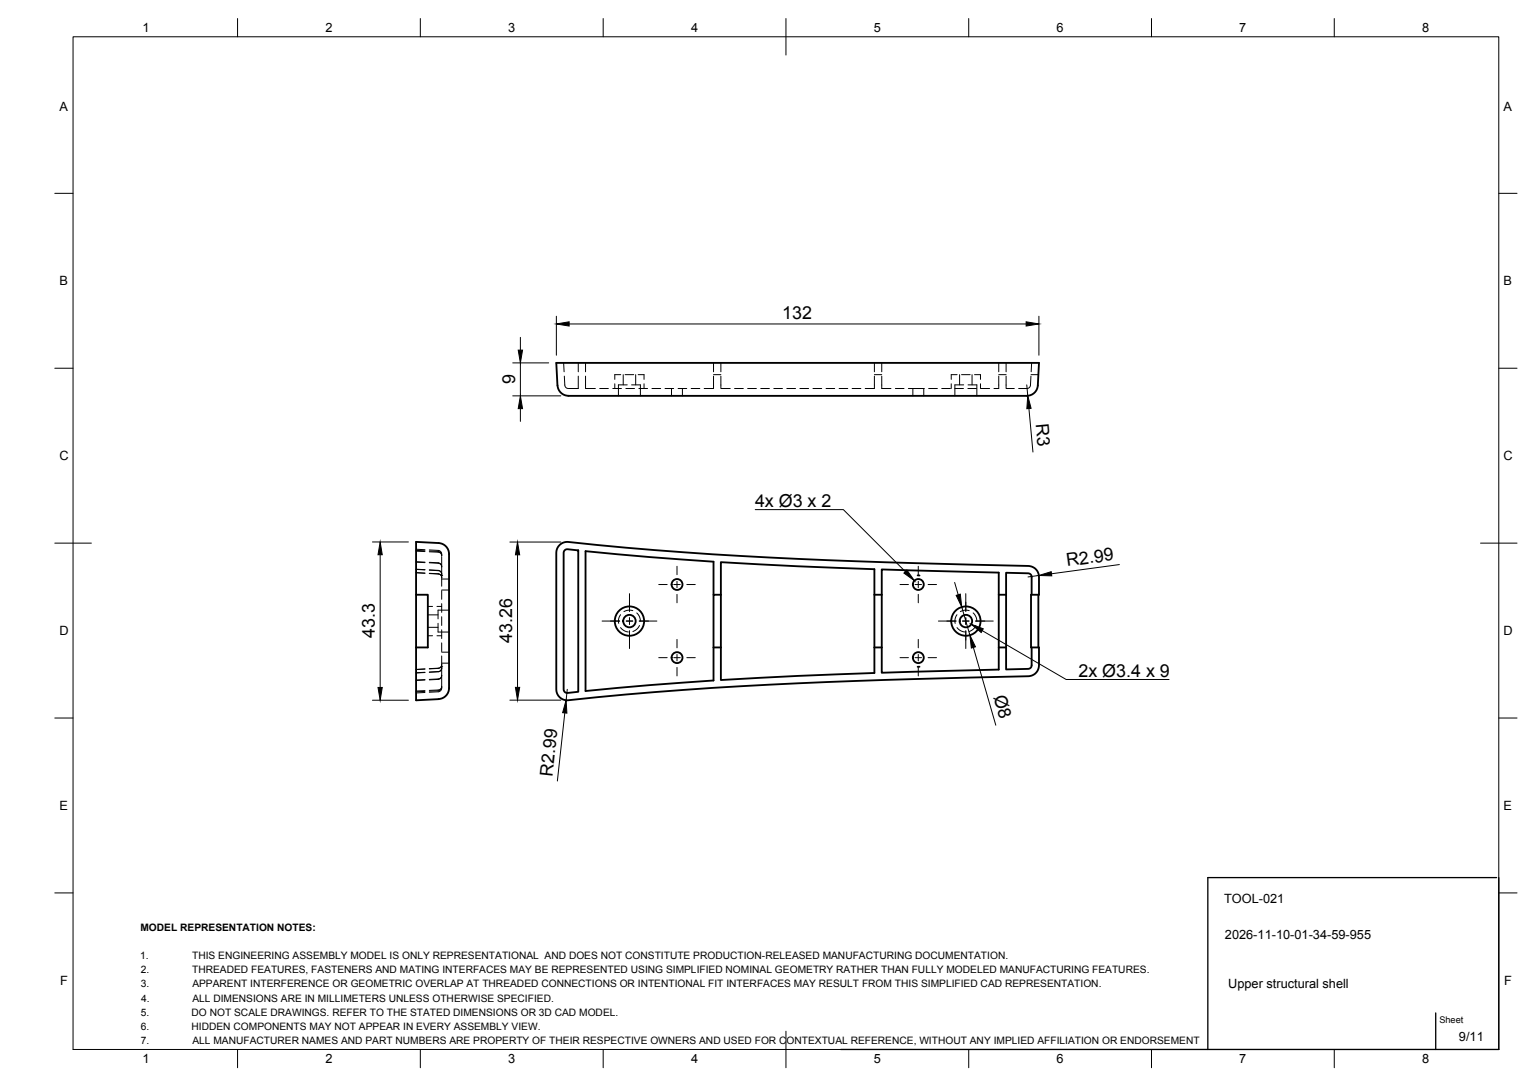
ISO-10303-21;
HEADER;
/* Generated by software containing ST-Developer
 * from STEP Tools, Inc. (www.steptools.com) 
 */

FILE_DESCRIPTION(
/* description */ (''),
/* implementation_level */ '2;1');

FILE_NAME(
/* name */ 'Upper structural shell.step',
/* time_stamp */ '2026-11-10T09:05:57-08:00',
/* author */ (''),
/* organization */ (''),
/* preprocessor_version */ 'ST-DEVELOPER v20.2',
/* originating_system */ 'Autodesk Translation Framework v15.17.0.0',
/* authorisation */ '');

FILE_SCHEMA (('AUTOMOTIVE_DESIGN { 1 0 10303 214 3 1 1 }'));
ENDSEC;

DATA;
#10=MECHANICAL_DESIGN_GEOMETRIC_PRESENTATION_REPRESENTATION('',(#569),#19618);
#75=SPHERICAL_SURFACE('',#7438,0.0999999999999999);
#76=SPHERICAL_SURFACE('',#7441,0.0999999999999997);
#77=SPHERICAL_SURFACE('',#7445,0.0999999999999998);
#78=SPHERICAL_SURFACE('',#7449,0.1);
#79=SPHERICAL_SURFACE('',#7454,0.3);
#80=SPHERICAL_SURFACE('',#7458,0.3);
#81=SPHERICAL_SURFACE('',#7462,0.3);
#82=SPHERICAL_SURFACE('',#7467,0.3);
#91=B_SPLINE_SURFACE_WITH_KNOTS('',3,3,((#10711,#10712,#10713,#10714),(#10715,
#10716,#10717,#10718),(#10719,#10720,#10721,#10722),(#10723,#10724,#10725,
#10726)),.UNSPECIFIED.,.F.,.F.,.F.,(4,4),(4,4),(0.0600191787356395,0.326709122771036),
(0.0105314009467253,0.683686938235975),.UNSPECIFIED.);
#92=B_SPLINE_SURFACE_WITH_KNOTS('',3,3,((#10731,#10732,#10733,#10734),(#10735,
#10736,#10737,#10738),(#10739,#10740,#10741,#10742),(#10743,#10744,#10745,
#10746)),.UNSPECIFIED.,.F.,.F.,.F.,(4,4),(4,4),(0.0251675824878611,0.0470055662028096),
(0.0103663370325175,0.682341693918943),.UNSPECIFIED.);
#93=B_SPLINE_SURFACE_WITH_KNOTS('',3,3,((#10756,#10757,#10758,#10759),(#10760,
#10761,#10762,#10763),(#10764,#10765,#10766,#10767),(#10768,#10769,#10770,
#10771),(#10772,#10773,#10774,#10775)),.UNSPECIFIED.,.F.,.F.,.F.,(4,1,4),
(4,4),(0.,0.571428571428571,1.),(0.796205213256333,4.31873271634551),
 .UNSPECIFIED.);
#94=B_SPLINE_SURFACE_WITH_KNOTS('',3,3,((#10780,#10781,#10782,#10783),(#10784,
#10785,#10786,#10787),(#10788,#10789,#10790,#10791),(#10792,#10793,#10794,
#10795),(#10796,#10797,#10798,#10799)),.UNSPECIFIED.,.F.,.F.,.F.,(4,1,4),
(4,4),(0.,0.571428571428571,1.),(0.335767855111383,0.605460332260614),
 .UNSPECIFIED.);
#95=B_SPLINE_SURFACE_WITH_KNOTS('',3,3,((#10818,#10819,#10820,#10821),(#10822,
#10823,#10824,#10825),(#10826,#10827,#10828,#10829),(#10830,#10831,#10832,
#10833),(#10834,#10835,#10836,#10837)),.UNSPECIFIED.,.F.,.F.,.F.,(4,1,4),
(4,4),(0.,0.571428571428571,1.),(8.8675541747208,12.3900816778099),
 .UNSPECIFIED.);
#96=B_SPLINE_SURFACE_WITH_KNOTS('',3,3,((#10842,#10843,#10844,#10845),(#10846,
#10847,#10848,#10849),(#10850,#10851,#10852,#10853),(#10854,#10855,#10856,
#10857)),.UNSPECIFIED.,.F.,.F.,.F.,(4,4),(4,4),(0.673290877228964,0.939980821264432),
(0.010531400969624,0.683686938235975),.UNSPECIFIED.);
#97=B_SPLINE_SURFACE_WITH_KNOTS('',3,3,((#10858,#10859,#10860,#10861),(#10862,
#10863,#10864,#10865),(#10866,#10867,#10868,#10869),(#10870,#10871,#10872,
#10873)),.UNSPECIFIED.,.F.,.F.,.F.,(4,4),(4,4),(0.952994433797115,0.974832417512139),
(0.0103663370325174,0.682341693895801),.UNSPECIFIED.);
#98=B_SPLINE_SURFACE_WITH_KNOTS('',3,3,((#10957,#10958,#10959,#10960),(#10961,
#10962,#10963,#10964),(#10965,#10966,#10967,#10968),(#10969,#10970,#10971,
#10972)),.UNSPECIFIED.,.F.,.F.,.F.,(4,4),(4,4),(0.341076481775573,0.660379921919131),
(0.0113804342297301,0.684288445414502),.UNSPECIFIED.);
#99=B_SPLINE_SURFACE_WITH_KNOTS('',3,3,((#10977,#10978,#10979,#10980),(#10981,
#10982,#10983,#10984),(#10985,#10986,#10987,#10988),(#10989,#10990,#10991,
#10992),(#10993,#10994,#10995,#10996)),.UNSPECIFIED.,.F.,.F.,.F.,(4,1,4),
(4,4),(0.,0.571428571428571,1.),(4.5128966022766,8.72381854299666),
 .UNSPECIFIED.);
#100=B_SPLINE_SURFACE_WITH_KNOTS('',3,3,((#11006,#11007,#11008,#11009),
(#11010,#11011,#11012,#11013),(#11014,#11015,#11016,#11017),(#11018,#11019,
#11020,#11021),(#11022,#11023,#11024,#11025)),.UNSPECIFIED.,.F.,.F.,.F.,
(4,1,4),(4,4),(0.,0.571428571428571,1.),(4.46246834806959,8.67339028878965),
 .UNSPECIFIED.);
#101=B_SPLINE_SURFACE_WITH_KNOTS('',3,3,((#11030,#11031,#11032,#11033),
(#11034,#11035,#11036,#11037),(#11038,#11039,#11040,#11041),(#11042,#11043,
#11044,#11045)),.UNSPECIFIED.,.F.,.F.,.F.,(4,4),(4,4),(0.33962007808087,
0.658923518224427),(0.0113804342297301,0.68428844541339),.UNSPECIFIED.);
#102=B_SPLINE_SURFACE_WITH_KNOTS('',3,3,((#11117,#11118,#11119,#11120),
(#11121,#11122,#11123,#11124),(#11125,#11126,#11127,#11128),(#11129,#11130,
#11131,#11132)),.UNSPECIFIED.,.F.,.F.,.F.,(4,4),(4,4),(0.67474627241906,
0.91907102854965),(0.0117551961069005,0.684448842095107),.UNSPECIFIED.);
#103=B_SPLINE_SURFACE_WITH_KNOTS('',3,3,((#11137,#11138,#11139,#11140),
(#11141,#11142,#11143,#11144),(#11145,#11146,#11147,#11148),(#11149,#11150,
#11151,#11152),(#11153,#11154,#11155,#11156)),.UNSPECIFIED.,.F.,.F.,.F.,
(4,1,4),(4,4),(0.,0.571428571428571,1.),(8.92068531110742,12.1251256661408),
 .UNSPECIFIED.);
#104=B_SPLINE_SURFACE_WITH_KNOTS('',3,3,((#11157,#11158,#11159,#11160),
(#11161,#11162,#11163,#11164),(#11165,#11166,#11167,#11168),(#11169,#11170,
#11171,#11172),(#11173,#11174,#11175,#11176)),.UNSPECIFIED.,.F.,.F.,.F.,
(4,1,4),(4,4),(0.,0.571428571428571,1.),(1.06116122492545,4.26560157995882),
 .UNSPECIFIED.);
#105=B_SPLINE_SURFACE_WITH_KNOTS('',3,3,((#11181,#11182,#11183,#11184),
(#11185,#11186,#11187,#11188),(#11189,#11190,#11191,#11192),(#11193,#11194,
#11195,#11196)),.UNSPECIFIED.,.F.,.F.,.F.,(4,4),(4,4),(0.0809289714503497,
0.325253727580939),(0.011755196108102,0.684448842095106),.UNSPECIFIED.);
#106=B_SPLINE_SURFACE_WITH_KNOTS('',3,3,((#11271,#11272,#11273,#11274),
(#11275,#11276,#11277,#11278),(#11279,#11280,#11281,#11282),(#11283,#11284,
#11285,#11286)),.UNSPECIFIED.,.F.,.F.,.F.,(4,4),(4,4),(0.932204931312898,
0.977820042778932),(0.0118590921259657,0.68448768567755),.UNSPECIFIED.);
#107=B_SPLINE_SURFACE_WITH_KNOTS('',3,3,((#11296,#11297,#11298,#11299),
(#11300,#11301,#11302,#11303),(#11304,#11305,#11306,#11307),(#11308,#11309,
#11310,#11311),(#11312,#11313,#11314,#11315)),.UNSPECIFIED.,.F.,.F.,.F.,
(4,1,4),(4,4),(0.,0.571428571428571,1.),(12.3228618033436,12.893479658151),
 .UNSPECIFIED.);
#108=B_SPLINE_SURFACE_WITH_KNOTS('',3,3,((#11329,#11330,#11331,#11332),
(#11333,#11334,#11335,#11336),(#11337,#11338,#11339,#11340),(#11341,#11342,
#11343,#11344)),.UNSPECIFIED.,.F.,.F.,.F.,(4,4),(4,4),(0.0221799572210682,
0.0677950686870383),(0.0118590921467069,0.68448768567755),.UNSPECIFIED.);
#109=B_SPLINE_SURFACE_WITH_KNOTS('',3,3,((#11354,#11355,#11356,#11357),
(#11358,#11359,#11360,#11361),(#11362,#11363,#11364,#11365),(#11366,#11367,
#11368,#11369),(#11370,#11371,#11372,#11373)),.UNSPECIFIED.,.F.,.F.,.F.,
(4,1,4),(4,4),(0.,0.571428571428571,1.),(0.29280723291527,0.863425087722636),
 .UNSPECIFIED.);
#110=B_SPLINE_SURFACE_WITH_KNOTS('',3,3,((#11387,#11388,#11389,#11390),
(#11391,#11392,#11393,#11394),(#11395,#11396,#11397,#11398),(#11399,#11400,
#11401,#11402),(#11403,#11404,#11405,#11406)),.UNSPECIFIED.,.F.,.F.,.F.,
(4,1,4),(4,4),(0.,0.571428571428571,1.),(0.00866835330220971,0.617725317592517),
 .UNSPECIFIED.);
#111=B_SPLINE_SURFACE_WITH_KNOTS('',3,3,((#11413,#11414,#11415,#11416),
(#11417,#11418,#11419,#11420),(#11421,#11422,#11423,#11424),(#11425,#11426,
#11427,#11428),(#11429,#11430,#11431,#11432),(#11433,#11434,#11435,#11436)),
 .UNSPECIFIED.,.F.,.F.,.F.,(4,1,1,4),(4,4),(0.,0.285714285714286,0.571428571428571,
1.),(0.00654045782928703,0.615688454110788),.UNSPECIFIED.);
#112=B_SPLINE_SURFACE_WITH_KNOTS('',3,3,((#11441,#11442,#11443,#11444),
(#11445,#11446,#11447,#11448),(#11449,#11450,#11451,#11452),(#11453,#11454,
#11455,#11456),(#11457,#11458,#11459,#11460),(#11461,#11462,#11463,#11464)),
 .UNSPECIFIED.,.F.,.F.,.F.,(4,1,1,4),(4,4),(0.,0.285714285714286,0.571428571428571,
1.),(0.00659363931523289,0.615688454110787),.UNSPECIFIED.);
#113=B_SPLINE_SURFACE_WITH_KNOTS('',3,3,((#11469,#11470,#11471,#11472),
(#11473,#11474,#11475,#11476),(#11477,#11478,#11479,#11480),(#11481,#11482,
#11483,#11484),(#11485,#11486,#11487,#11488)),.UNSPECIFIED.,.F.,.F.,.F.,
(4,1,4),(4,4),(0.,0.571428571428571,1.),(12.5808265588057,12.8505190359549),
 .UNSPECIFIED.);
#114=B_SPLINE_SURFACE_WITH_KNOTS('',3,3,((#11489,#11490,#11491,#11492),
(#11493,#11494,#11495,#11496),(#11497,#11498,#11499,#11500),(#11501,#11502,
#11503,#11504),(#11505,#11506,#11507,#11508)),.UNSPECIFIED.,.F.,.F.,.F.,
(4,1,4),(4,4),(0.,0.571428571428571,1.),(0.00865878607617127,0.617725317592517),
 .UNSPECIFIED.);
#115=B_SPLINE_SURFACE_WITH_KNOTS('',3,3,((#11534,#11535,#11536,#11537),
(#11538,#11539,#11540,#11541),(#11542,#11543,#11544,#11545),(#11546,#11547,
#11548,#11549),(#11550,#11551,#11552,#11553)),.UNSPECIFIED.,.F.,.F.,.F.,
(4,1,4),(4,4),(0.,0.571428571428571,1.),(-0.00615755989250974,0.617725317592517),
 .UNSPECIFIED.);
#116=B_SPLINE_SURFACE_WITH_KNOTS('',3,3,((#11572,#11573,#11574,#11575,#11576),
(#11577,#11578,#11579,#11580,#11581),(#11582,#11583,#11584,#11585,#11586),
(#11587,#11588,#11589,#11590,#11591),(#11592,#11593,#11594,#11595,#11596)),
 .UNSPECIFIED.,.F.,.F.,.F.,(4,1,4),(4,1,4),(0.,0.571428571428571,1.),(0.335767855111383,
5.71764434212835,12.893479658151),.UNSPECIFIED.);
#117=B_SPLINE_SURFACE_WITH_KNOTS('',3,3,((#11607,#11608,#11609,#11610),
(#11611,#11612,#11613,#11614),(#11615,#11616,#11617,#11618),(#11619,#11620,
#11621,#11622),(#11623,#11624,#11625,#11626),(#11627,#11628,#11629,#11630)),
 .UNSPECIFIED.,.F.,.F.,.F.,(4,1,1,4),(4,4),(0.,0.285714285714286,0.571428571428571,
1.),(-0.00844595120920508,0.615688454110788),.UNSPECIFIED.);
#118=B_SPLINE_SURFACE_WITH_KNOTS('',3,3,((#11639,#11640,#11641,#11642),
(#11643,#11644,#11645,#11646),(#11647,#11648,#11649,#11650),(#11651,#11652,
#11653,#11654),(#11655,#11656,#11657,#11658),(#11659,#11660,#11661,#11662)),
 .UNSPECIFIED.,.F.,.F.,.F.,(4,1,1,4),(4,4),(0.,0.285714285714286,0.571428571428571,
1.),(-0.00828643285111643,0.615688454110787),.UNSPECIFIED.);
#119=B_SPLINE_SURFACE_WITH_KNOTS('',3,3,((#11671,#11672,#11673,#11674,#11675),
(#11676,#11677,#11678,#11679,#11680),(#11681,#11682,#11683,#11684,#11685),
(#11686,#11687,#11688,#11689,#11690),(#11691,#11692,#11693,#11694,#11695)),
 .UNSPECIFIED.,.F.,.F.,.F.,(4,1,4),(4,1,4),(0.,0.571428571428571,1.),(0.29280723291527,
7.4686425489379,12.8505190359549),.UNSPECIFIED.);
#120=B_SPLINE_SURFACE_WITH_KNOTS('',3,3,((#11706,#11707,#11708,#11709),
(#11710,#11711,#11712,#11713),(#11714,#11715,#11716,#11717),(#11718,#11719,
#11720,#11721),(#11722,#11723,#11724,#11725)),.UNSPECIFIED.,.F.,.F.,.F.,
(4,1,4),(4,4),(0.,0.571428571428571,1.),(-0.0061862132014275,0.617725317592517),
 .UNSPECIFIED.);
#121=B_SPLINE_SURFACE_WITH_KNOTS('',3,3,((#11734,#11735,#11736,#11737),
(#11738,#11739,#11740,#11741),(#11742,#11743,#11744,#11745),(#11746,#11747,
#11748,#11749)),.UNSPECIFIED.,.F.,.F.,.F.,(4,4),(4,4),(0.025165545222094,
0.977821881680028),(0.,0.68448768567755),.UNSPECIFIED.);
#122=B_SPLINE_SURFACE_WITH_KNOTS('',3,3,((#11752,#11753,#11754,#11755),
(#11756,#11757,#11758,#11759),(#11760,#11761,#11762,#11763),(#11764,#11765,
#11766,#11767)),.UNSPECIFIED.,.F.,.F.,.F.,(4,4),(4,4),(0.0221781183199723,
0.974834454777906),(0.,0.68448768567755),.UNSPECIFIED.);
#171=B_SPLINE_CURVE_WITH_KNOTS('',3,(#9725,#9726,#9727,#9728),
 .UNSPECIFIED.,.F.,.F.,(4,4),(3.28016616408593,4.26236080300681),
 .UNSPECIFIED.);
#172=B_SPLINE_CURVE_WITH_KNOTS('',3,(#9732,#9733,#9734,#9735),
 .UNSPECIFIED.,.F.,.F.,(4,4),(8.92392608805945,9.90612072688831),
 .UNSPECIFIED.);
#173=B_SPLINE_CURVE_WITH_KNOTS('',3,(#9737,#9738,#9739,#9740,#9741,#9742,
#9743,#9744,#9745,#9746,#9747,#9748,#9749,#9750,#9751,#9752,#9753,#9754,
#9755),.UNSPECIFIED.,.F.,.F.,(4,3,3,3,3,3,4),(-0.050768112872884,-0.0388528786649772,
-0.0311058171716578,-0.0259830388669653,-0.0210744122964195,-0.0143837148934404,
0.),.UNSPECIFIED.);
#174=B_SPLINE_CURVE_WITH_KNOTS('',3,(#9757,#9758,#9759,#9760),
 .UNSPECIFIED.,.F.,.F.,(4,4),(9.9568018127159,12.1251256661408),
 .UNSPECIFIED.);
#175=B_SPLINE_CURVE_WITH_KNOTS('',3,(#9764,#9765,#9766,#9767),
 .UNSPECIFIED.,.F.,.F.,(4,4),(1.06116122492545,3.22948508825557),
 .UNSPECIFIED.);
#176=B_SPLINE_CURVE_WITH_KNOTS('',3,(#9768,#9769,#9770,#9771,#9772,#9773,
#9774,#9775,#9776,#9777,#9778,#9779,#9780,#9781,#9782,#9783,#9784,#9785,
#9786),.UNSPECIFIED.,.F.,.F.,(4,3,3,3,3,3,4),(-0.0507681129736439,-0.0388528772897764,
-0.0311058147321604,-0.0259830361493327,-0.0210744097201194,-0.0143837130754026,
-9.90506278315E-9),.UNSPECIFIED.);
#177=B_SPLINE_CURVE_WITH_KNOTS('',3,(#9934,#9935,#9936,#9937,#9938,#9939),
 .UNSPECIFIED.,.F.,.F.,(4,2,4),(-0.605566356596631,-0.303329629920269,-0.000148729590407126),
 .UNSPECIFIED.);
#178=B_SPLINE_CURVE_WITH_KNOTS('',3,(#9941,#9942,#9943,#9944,#9945,#9946,
#9947,#9948,#9949,#9950,#9951,#9952,#9953,#9954,#9955,#9956,#9957,#9958,
#9959,#9960,#9961,#9962,#9963,#9964,#9965,#9966,#9967,#9968),
 .UNSPECIFIED.,.F.,.F.,(4,3,3,3,3,3,3,3,3,4),(-0.153210533292091,-0.129383071834804,
-0.117098895005168,-0.0931297672424715,-0.0778761857300216,-0.065564095006876,
-0.0417435583396367,-0.038874550231651,-0.0150983388519663,0.),
 .UNSPECIFIED.);
#179=B_SPLINE_CURVE_WITH_KNOTS('',3,(#9972,#9973,#9974,#9975,#9976,#9977,
#9978,#9979,#9980,#9981,#9982,#9983,#9984,#9985,#9986,#9987,#9988,#9989,
#9990,#9991,#9992,#9993,#9994,#9995,#9996,#9997,#9998,#9999),
 .UNSPECIFIED.,.F.,.F.,(4,3,3,3,3,3,3,3,3,4),(-0.153244081227051,-0.129493605146206,
-0.117970006482883,-0.0941492904140308,-0.0876825809854227,-0.078828741443105,
-0.0548877675055393,-0.0394694906046094,-0.0155984926894347,0.),
 .UNSPECIFIED.);
#180=B_SPLINE_CURVE_WITH_KNOTS('',3,(#10000,#10001,#10002,#10003,#10004,
#10005),.UNSPECIFIED.,.F.,.F.,(4,2,4),(-0.606539490527658,-0.303329031627741,
-0.00112184825655631),.UNSPECIFIED.);
#181=B_SPLINE_CURVE_WITH_KNOTS('',3,(#10010,#10011,#10012,#10013,#10014,
#10015),.UNSPECIFIED.,.F.,.F.,(4,2,4),(-0.606785247764818,-0.303663188081886,
-0.00088649083675002),.UNSPECIFIED.);
#182=B_SPLINE_CURVE_WITH_KNOTS('',3,(#10017,#10018,#10019,#10020,#10021,
#10022,#10023,#10024,#10025,#10026,#10027,#10028,#10029,#10030,#10031,#10032,
#10033,#10034,#10035,#10036,#10037,#10038,#10039,#10040,#10041,#10042,#10043,
#10044),.UNSPECIFIED.,.F.,.F.,(4,3,3,3,3,3,3,3,3,4),(-0.15258577077829,
-0.128839317352572,-0.117158786685373,-0.0932148261566644,-0.0780319390000633,
-0.0653676349965338,-0.0415665498371782,-0.0389909618069961,-0.0152059030050533,
0.),.UNSPECIFIED.);
#183=B_SPLINE_CURVE_WITH_KNOTS('',3,(#10048,#10049,#10050,#10051,#10052,
#10053,#10054,#10055,#10056,#10057,#10058,#10059,#10060,#10061,#10062,#10063,
#10064,#10065,#10066,#10067,#10068,#10069,#10070,#10071,#10072,#10073,#10074,
#10075),.UNSPECIFIED.,.F.,.F.,(4,3,3,3,3,3,3,3,3,4),(-0.152596853546747,
-0.128825864440686,-0.115507515430042,-0.0917263797372463,-0.0872428123353572,
-0.0783995504057471,-0.0544835945915644,-0.0392209901554083,-0.0154275313391792,
0.),.UNSPECIFIED.);
#184=B_SPLINE_CURVE_WITH_KNOTS('',3,(#10077,#10078,#10079,#10080,#10081,
#10082),.UNSPECIFIED.,.F.,.F.,(4,2,4),(-0.606440835737524,-0.303663090452391,
-0.000542069086802599),.UNSPECIFIED.);
#185=B_SPLINE_CURVE_WITH_KNOTS('',3,(#10088,#10089,#10090,#10091,#10092,
#10093),.UNSPECIFIED.,.F.,.F.,(4,2,4),(-0.607379220946441,-0.303761646676304,
-0.00124422999587004),.UNSPECIFIED.);
#186=B_SPLINE_CURVE_WITH_KNOTS('',3,(#10095,#10096,#10097,#10098,#10099,
#10100,#10101,#10102,#10103,#10104,#10105,#10106,#10107,#10108,#10109,#10110,
#10111,#10112,#10113,#10114,#10115,#10116,#10117,#10118,#10119,#10120,#10121,
#10122),.UNSPECIFIED.,.F.,.F.,(4,3,3,3,3,3,3,3,3,4),(-0.152287640102895,
-0.128554450486317,-0.115193035178751,-0.0912770810520543,-0.0781028969167454,
-0.0652733399726575,-0.0414820896655672,-0.0390446621366508,-0.0152552334863041,
0.),.UNSPECIFIED.);
#187=B_SPLINE_CURVE_WITH_KNOTS('',3,(#10126,#10127,#10128,#10129,#10130,
#10131,#10132,#10133,#10134,#10135,#10136,#10137,#10138,#10139,#10140,#10141,
#10142,#10143,#10144,#10145,#10146,#10147,#10148,#10149,#10150,#10151,#10152,
#10153),.UNSPECIFIED.,.F.,.F.,(4,3,3,3,3,3,3,3,3,4),(-0.152291020205185,
-0.128517753946702,-0.115248901231919,-0.0914807886786037,-0.0870359119466785,
-0.0782017654295232,-0.054298407767766,-0.03910658747416,-0.0153486482327859,
0.),.UNSPECIFIED.);
#188=B_SPLINE_CURVE_WITH_KNOTS('',3,(#10155,#10156,#10157,#10158,#10159,
#10160),.UNSPECIFIED.,.F.,.F.,(4,2,4),(-0.606279550122448,-0.303761677523001,
-0.000144559171857295),.UNSPECIFIED.);
#189=B_SPLINE_CURVE_WITH_KNOTS('',3,(#10166,#10167,#10168,#10169,#10170,
#10171),.UNSPECIFIED.,.F.,.F.,(4,2,4),(-0.607536685592867,-0.303784463250135,
-0.00133982193348342),.UNSPECIFIED.);
#190=B_SPLINE_CURVE_WITH_KNOTS('',3,(#10172,#10173,#10174,#10175,#10176,
#10177,#10178,#10179,#10180,#10181,#10182,#10183,#10184,#10185,#10186,#10187,
#10188,#10189,#10190,#10191,#10192,#10193,#10194,#10195,#10196,#10197,#10198,
#10199),.UNSPECIFIED.,.F.,.F.,(4,3,3,3,3,3,3,3,3,4),(-0.152217684890348,
-0.128490376540845,-0.11516578527262,-0.091253137134092,-0.0781160865160423,
-0.0652495101170982,-0.0414606291875136,-0.0390546905501479,-0.015263466236765,
0.),.UNSPECIFIED.);
#191=B_SPLINE_CURVE_WITH_KNOTS('',3,(#10201,#10202,#10203,#10204,#10205,
#10206,#10207,#10208,#10209,#10210,#10211,#10212,#10213,#10214,#10215,#10216,
#10217,#10218,#10219,#10220,#10221,#10222,#10223,#10224,#10225,#10226,#10227,
#10228),.UNSPECIFIED.,.F.,.F.,(4,3,3,3,3,3,3,3,3,4),(-0.152219351639196,
-0.128444680332832,-0.115193337419806,-0.0914284185691762,-0.0869890032859244,
-0.0781648487722283,-0.0542647883944502,-0.0390852411900305,-0.0153331469286526,
0.),.UNSPECIFIED.);
#192=B_SPLINE_CURVE_WITH_KNOTS('',3,(#10230,#10231,#10232,#10233,#10234,
#10235),.UNSPECIFIED.,.F.,.F.,(4,2,4),(-0.606231877025315,-0.303784501204342,
-3.50089943914611E-5),.UNSPECIFIED.);
#193=B_SPLINE_CURVE_WITH_KNOTS('',3,(#10241,#10242,#10243,#10244),
 .UNSPECIFIED.,.F.,.F.,(4,4),(0.0108333608245492,0.617725317592517),
 .UNSPECIFIED.);
#194=B_SPLINE_CURVE_WITH_KNOTS('',3,(#10248,#10249,#10250,#10251),
 .UNSPECIFIED.,.F.,.F.,(4,4),(-0.617725317592517,-0.0108333608245492),
 .UNSPECIFIED.);
#195=B_SPLINE_CURVE_WITH_KNOTS('',3,(#10254,#10255,#10256,#10257),
 .UNSPECIFIED.,.F.,.F.,(4,4),(8.65483889175297,12.1899094612697),
 .UNSPECIFIED.);
#196=B_SPLINE_CURVE_WITH_KNOTS('',3,(#10258,#10259,#10260,#10261),
 .UNSPECIFIED.,.F.,.F.,(4,4),(0.491886782059505,4.00844302274363),
 .UNSPECIFIED.);
#197=B_SPLINE_CURVE_WITH_KNOTS('',3,(#10264,#10265,#10266,#10267,#10268,
#10269,#10270,#10271,#10272,#10273),.UNSPECIFIED.,.F.,.F.,(4,3,3,4),(4.20909064274042,
6.3236533433415,8.26419514194387,8.41669725637478),.UNSPECIFIED.);
#198=B_SPLINE_CURVE_WITH_KNOTS('',3,(#10276,#10277,#10278,#10279),
 .UNSPECIFIED.,.F.,.F.,(4,4),(8.61714174069208,11.8187712274298),
 .UNSPECIFIED.);
#199=B_SPLINE_CURVE_WITH_KNOTS('',3,(#10283,#10284,#10285,#10286),
 .UNSPECIFIED.,.F.,.F.,(4,4),(12.0182076143484,12.6179302061492),
 .UNSPECIFIED.);
#200=B_SPLINE_CURVE_WITH_KNOTS('',3,(#10287,#10288,#10289,#10290,#10291,
#10292,#10293,#10294,#10295,#10296,#10297,#10298,#10299,#10300,#10301,#10302,
#10303,#10304,#10305,#10306,#10307,#10308,#10309,#10310,#10311,#10312,#10313,
#10314),.UNSPECIFIED.,.F.,.F.,(4,3,3,3,3,3,3,3,3,4),(0.,0.023812730958415,
0.0390943730497349,0.0628727645281949,0.0664866407211859,0.0780895647789142,
0.102003044086093,0.117056568347941,0.14081843048439,0.155095961761698),
 .UNSPECIFIED.);
#201=B_SPLINE_CURVE_WITH_KNOTS('',3,(#10318,#10319,#10320,#10321,#10322,
#10323,#10324,#10325,#10326,#10327,#10328,#10329,#10330,#10331,#10332,#10333,
#10334,#10335,#10336,#10337,#10338,#10339,#10340,#10341,#10342,#10343,#10344,
#10345,#10346,#10347,#10348,#10349,#10350,#10351,#10352,#10353,#10354),
 .UNSPECIFIED.,.F.,.F.,(4,3,3,3,3,3,3,3,3,3,3,3,4),(0.,0.0535193130531386,
0.107740084455895,0.117281563739951,0.171478196787188,0.199460035548543,
0.234266327019636,0.287962832542679,0.34249270416273,0.351167719367162,
0.408228095477446,0.46132246935065,0.46528847158773),.UNSPECIFIED.);
#202=B_SPLINE_CURVE_WITH_KNOTS('',3,(#10356,#10357,#10358,#10359),
 .UNSPECIFIED.,.F.,.F.,(4,4),(0.0221781183199723,0.974834454777906),
 .UNSPECIFIED.);
#203=B_SPLINE_CURVE_WITH_KNOTS('',3,(#10361,#10362,#10363,#10364,#10365,
#10366,#10367,#10368,#10369,#10370,#10371,#10372,#10373,#10374,#10375,#10376,
#10377,#10378,#10379,#10380,#10381,#10382,#10383,#10384,#10385,#10386,#10387,
#10388,#10389,#10390,#10391,#10392,#10393,#10394,#10395,#10396,#10397,#10398,
#10399,#10400,#10401,#10402,#10403),.UNSPECIFIED.,.F.,.F.,(4,3,3,3,3,3,
3,3,3,3,3,3,3,3,4),(0.,0.0533317239385299,0.107762434368039,0.117305236535198,
0.171635266834242,0.216430402805854,0.234303130921432,0.288010415584935,
0.341932185058889,0.351200358601802,0.360578786332496,0.414653942238971,
0.427906071157934,0.482008506259547,0.504658879840573),.UNSPECIFIED.);
#204=B_SPLINE_CURVE_WITH_KNOTS('',3,(#10407,#10408,#10409,#10410,#10411,
#10412,#10413,#10414,#10415,#10416,#10417,#10418,#10419,#10420,#10421,#10422,
#10423,#10424,#10425,#10426,#10427,#10428,#10429,#10430,#10431,#10432,#10433,
#10434,#10435,#10436,#10437,#10438,#10439,#10440,#10441,#10442,#10443,#10444,
#10445,#10446,#10447,#10448,#10449),.UNSPECIFIED.,.F.,.F.,(4,3,3,3,3,3,
3,3,3,3,3,3,3,3,4),(0.,0.0533492049661439,0.107791770949794,0.117401360885473,
0.171729175646356,0.216477851539682,0.234467324023732,0.288191829779795,
0.342104640447882,0.351366010290958,0.360619117109406,0.414688080797906,
0.427993719046535,0.482081475021072,0.504664253934307),.UNSPECIFIED.);
#205=B_SPLINE_CURVE_WITH_KNOTS('',3,(#10451,#10452,#10453,#10454),
 .UNSPECIFIED.,.F.,.F.,(4,4),(0.0251655452220943,0.977821881680028),
 .UNSPECIFIED.);
#206=B_SPLINE_CURVE_WITH_KNOTS('',3,(#10456,#10457,#10458,#10459,#10460,
#10461,#10462,#10463,#10464,#10465,#10466,#10467,#10468,#10469,#10470,#10471,
#10472,#10473,#10474,#10475,#10476,#10477,#10478,#10479,#10480,#10481,#10482,
#10483,#10484,#10485,#10486,#10487,#10488,#10489,#10490,#10491,#10492),
 .UNSPECIFIED.,.F.,.F.,(4,3,3,3,3,3,3,3,3,3,3,3,4),(0.,0.053523079491772,
0.107745541051727,0.117301531762597,0.171497090450284,0.19946878868074,
0.234298606923062,0.287998861062908,0.34252758042597,0.351197710209308,
0.408243668718811,0.4613343165756,0.465289627228313),.UNSPECIFIED.);
#207=B_SPLINE_CURVE_WITH_KNOTS('',3,(#10495,#10496,#10497,#10498,#10499,
#10500,#10501,#10502,#10503,#10504,#10505,#10506,#10507,#10508,#10509,#10510,
#10511,#10512,#10513,#10514,#10515,#10516,#10517,#10518,#10519,#10520,#10521,
#10522),.UNSPECIFIED.,.F.,.F.,(4,3,3,3,3,3,3,3,3,4),(0.,0.0238139464176845,
0.039101051769884,0.0628789982206146,0.0664894862143964,0.0781003874493316,
0.102014483019035,0.11706667068295,0.140827139970411,0.155096347075245),
 .UNSPECIFIED.);
#208=B_SPLINE_CURVE_WITH_KNOTS('',3,(#10524,#10525,#10526,#10527),
 .UNSPECIFIED.,.F.,.F.,(4,4),(2.42791692093292E-5,0.602904494019558),
 .UNSPECIFIED.);
#209=B_SPLINE_CURVE_WITH_KNOTS('',3,(#10530,#10531,#10532,#10533),
 .UNSPECIFIED.,.F.,.F.,(4,4),(0.8033909285608,4.02187648095927),
 .UNSPECIFIED.);
#210=B_SPLINE_CURVE_WITH_KNOTS('',3,(#10536,#10537,#10538,#10539,#10540,
#10541,#10542,#10543,#10544,#10545),.UNSPECIFIED.,.F.,.F.,(4,3,3,4),(4.22337623295021,
6.17414866693447,6.32726315261627,8.45313487255185),.UNSPECIFIED.);
#211=B_SPLINE_CURVE_WITH_KNOTS('',3,(#10549,#10550,#10551,#10552),
 .UNSPECIFIED.,.F.,.F.,(4,4),(12.3921295467468,12.6843586902602),
 .UNSPECIFIED.);
#212=B_SPLINE_CURVE_WITH_KNOTS('',3,(#10554,#10555,#10556,#10557,#10558,
#10559,#10560,#10561,#10562,#10563,#10564,#10565,#10566,#10567,#10568,#10569,
#10570,#10571,#10572,#10573,#10574,#10575,#10576,#10577,#10578,#10579,#10580,
#10581,#10582,#10583,#10584,#10585,#10586,#10587),.UNSPECIFIED.,.F.,.F.,
(4,3,3,3,3,3,3,3,3,3,3,4),(0.,0.0238043957114055,0.0391346151758438,0.0629652053320384,
0.0721593756253901,0.0781571886687045,0.101948185591131,0.117123476992186,
0.12020682003633,0.142665945482357,0.166389927689249,0.168222194312373),
 .UNSPECIFIED.);
#213=B_SPLINE_CURVE_WITH_KNOTS('',3,(#10591,#10592,#10593,#10594,#10595,
#10596,#10597,#10598,#10599,#10600,#10601,#10602,#10603,#10604,#10605,#10606,
#10607,#10608,#10609,#10610,#10611,#10612,#10613,#10614,#10615,#10616,#10617,
#10618,#10619,#10620,#10621,#10622,#10623,#10624),.UNSPECIFIED.,.F.,.F.,
(4,3,3,3,3,3,3,3,3,3,3,4),(0.,0.023797882907907,0.039102479174454,0.0629340675289177,
0.0721439954475325,0.0781021576199648,0.101891255326939,0.117067721419617,
0.120193732390416,0.142636523050355,0.16636673084783,0.168220399847748),
 .UNSPECIFIED.);
#214=B_SPLINE_CURVE_WITH_KNOTS('',3,(#10626,#10627,#10628,#10629),
 .UNSPECIFIED.,.F.,.F.,(4,4),(2.71213177756024E-5,0.290725780256064),
 .UNSPECIFIED.);
#215=B_SPLINE_CURVE_WITH_KNOTS('',3,(#10639,#10640,#10641,#10642,#10643,
#10644),.UNSPECIFIED.,.F.,.F.,(4,2,4),(-0.6065913737563,-0.303324265158378,
-0.00121210420063977),.UNSPECIFIED.);
#216=B_SPLINE_CURVE_WITH_KNOTS('',3,(#10646,#10647,#10648,#10649,#10650,
#10651),.UNSPECIFIED.,.F.,.F.,(4,2,4),(-0.605468679705391,-0.303324901248498,
-8.9425867424664E-5),.UNSPECIFIED.);
#217=B_SPLINE_CURVE_WITH_KNOTS('',3,(#10653,#10654,#10655,#10656,#10657,
#10658,#10659,#10660,#10661,#10662,#10663,#10664,#10665,#10666,#10667,#10668,
#10669,#10670,#10671,#10672,#10673,#10674,#10675,#10676,#10677,#10678,#10679,
#10680),.UNSPECIFIED.,.F.,.F.,(4,3,3,3,3,3,3,3,3,4),(-0.153261590805415,
-0.129427422483982,-0.117093626371441,-0.093122524304512,-0.077863059046492,
-0.0655799937729104,-0.0417579003169496,-0.0388648221790391,-0.0150894148558222,
0.),.UNSPECIFIED.);
#218=B_SPLINE_CURVE_WITH_KNOTS('',3,(#10683,#10684,#10685,#10686,#10687,
#10688,#10689,#10690,#10691,#10692,#10693,#10694,#10695,#10696,#10697,#10698,
#10699,#10700,#10701,#10702,#10703,#10704,#10705,#10706,#10707,#10708,#10709,
#10710),.UNSPECIFIED.,.F.,.F.,(4,3,3,3,3,3,3,3,3,4),(-0.153296867786173,
-0.129546774976449,-0.118009772088948,-0.0941871764575653,-0.08771862273971,
-0.0788646444725944,-0.0549216410880561,-0.0394902966566095,-0.0156128557692252,
0.),.UNSPECIFIED.);
#219=B_SPLINE_CURVE_WITH_KNOTS('',3,(#10727,#10728,#10729,#10730),
 .UNSPECIFIED.,.F.,.F.,(4,4),(-4.3123055228435,-0.796205213256333),
 .UNSPECIFIED.);
#220=B_SPLINE_CURVE_WITH_KNOTS('',3,(#10748,#10749,#10750,#10751),
 .UNSPECIFIED.,.F.,.F.,(4,4),(-0.594853877716395,-0.335767855111383),
 .UNSPECIFIED.);
#221=B_SPLINE_CURVE_WITH_KNOTS('',3,(#10752,#10753,#10754,#10755),
 .UNSPECIFIED.,.F.,.F.,(4,4),(-0.615688454110788,-0.00935595183171186),
 .UNSPECIFIED.);
#222=B_SPLINE_CURVE_WITH_KNOTS('',3,(#10776,#10777,#10778,#10779),
 .UNSPECIFIED.,.F.,.F.,(4,4),(0.806548880270408,4.31873271634551),
 .UNSPECIFIED.);
#223=B_SPLINE_CURVE_WITH_KNOTS('',3,(#10801,#10802,#10803,#10804),
 .UNSPECIFIED.,.F.,.F.,(4,4),(0.335767855111383,0.605460332260614),
 .UNSPECIFIED.);
#224=B_SPLINE_CURVE_WITH_KNOTS('',3,(#10807,#10808,#10809,#10810),
 .UNSPECIFIED.,.F.,.F.,(4,4),(8.8675541747208,12.379738010796),
 .UNSPECIFIED.);
#225=B_SPLINE_CURVE_WITH_KNOTS('',3,(#10813,#10814,#10815,#10816),
 .UNSPECIFIED.,.F.,.F.,(4,4),(12.5808265588057,12.8505190359549),
 .UNSPECIFIED.);
#226=B_SPLINE_CURVE_WITH_KNOTS('',3,(#10838,#10839,#10840,#10841),
 .UNSPECIFIED.,.F.,.F.,(4,4),(-12.3900816778099,-8.87398136822274),
 .UNSPECIFIED.);
#227=B_SPLINE_CURVE_WITH_KNOTS('',3,(#10875,#10876,#10877,#10878),
 .UNSPECIFIED.,.F.,.F.,(4,4),(0.00935595183171174,0.615688454110787),
 .UNSPECIFIED.);
#228=B_SPLINE_CURVE_WITH_KNOTS('',3,(#10879,#10880,#10881,#10882),
 .UNSPECIFIED.,.F.,.F.,(4,4),(-12.8505190359549,-12.5914330133498),
 .UNSPECIFIED.);
#229=B_SPLINE_CURVE_WITH_KNOTS('',3,(#10885,#10886,#10887,#10888,#10889,
#10890),.UNSPECIFIED.,.F.,.F.,(4,2,4),(-0.606830654194234,-0.303665168982051,
-0.00091389508118378),.UNSPECIFIED.);
#230=B_SPLINE_CURVE_WITH_KNOTS('',3,(#10892,#10893,#10894,#10895,#10896,
#10897,#10898,#10899,#10900,#10901,#10902,#10903,#10904,#10905,#10906,#10907,
#10908,#10909,#10910,#10911,#10912,#10913,#10914,#10915,#10916,#10917,#10918,
#10919),.UNSPECIFIED.,.F.,.F.,(4,3,3,3,3,3,3,3,3,4),(-0.152562937837783,
-0.12881903955137,-0.117160811640917,-0.0932181166800446,-0.0780374575565173,
-0.0653603882662585,-0.0415602279441365,-0.0389951227734853,-0.0152093108541457,
0.),.UNSPECIFIED.);
#231=B_SPLINE_CURVE_WITH_KNOTS('',3,(#10923,#10924,#10925,#10926,#10927,
#10928,#10929,#10930,#10931,#10932,#10933,#10934,#10935,#10936,#10937,#10938,
#10939,#10940,#10941,#10942,#10943,#10944,#10945,#10946,#10947,#10948,#10949,
#10950),.UNSPECIFIED.,.F.,.F.,(4,3,3,3,3,3,3,3,3,4),(-0.152573286042523,
-0.128801685906155,-0.115487540236632,-0.091707628219999,-0.0872268515824704,
-0.07838422198738,-0.0544695788315335,-0.0392121213631617,-0.0154211067806385,
0.),.UNSPECIFIED.);
#232=B_SPLINE_CURVE_WITH_KNOTS('',3,(#10951,#10952,#10953,#10954,#10955,
#10956),.UNSPECIFIED.,.F.,.F.,(4,2,4),(-0.606417229744719,-0.30366508312326,
-0.000500462001714608),.UNSPECIFIED.);
#233=B_SPLINE_CURVE_WITH_KNOTS('',3,(#10973,#10974,#10975,#10976),
 .UNSPECIFIED.,.F.,.F.,(4,4),(-8.7204856127415,-4.5128966022766),
 .UNSPECIFIED.);
#234=B_SPLINE_CURVE_WITH_KNOTS('',3,(#10997,#10998,#10999,#11000),
 .UNSPECIFIED.,.F.,.F.,(4,4),(4.51913891174751,8.72381854299666),
 .UNSPECIFIED.);
#235=B_SPLINE_CURVE_WITH_KNOTS('',3,(#11002,#11003,#11004,#11005),
 .UNSPECIFIED.,.F.,.F.,(4,4),(4.46246834806959,8.66714797931881),
 .UNSPECIFIED.);
#236=B_SPLINE_CURVE_WITH_KNOTS('',3,(#11026,#11027,#11028,#11029),
 .UNSPECIFIED.,.F.,.F.,(4,4),(-8.67339028878965,-4.46580127832475),
 .UNSPECIFIED.);
#237=B_SPLINE_CURVE_WITH_KNOTS('',3,(#11048,#11049,#11050,#11051,#11052,
#11053),.UNSPECIFIED.,.F.,.F.,(4,2,4),(-0.607391644691745,-0.303762155877002,
-0.00125172564267001),.UNSPECIFIED.);
#238=B_SPLINE_CURVE_WITH_KNOTS('',3,(#11054,#11055,#11056,#11057,#11058,
#11059,#11060,#11061,#11062,#11063,#11064,#11065,#11066,#11067,#11068,#11069,
#11070,#11071,#11072,#11073,#11074,#11075,#11076,#11077,#11078,#11079,#11080,
#11081),.UNSPECIFIED.,.F.,.F.,(4,3,3,3,3,3,3,3,3,4),(-0.152281539067936,
-0.12854821222061,-0.115190816126163,-0.0912758856104041,-0.0781043161616985,
-0.0652713841318381,-0.0414808619979686,-0.039045740680325,-0.0152551599791835,
0.),.UNSPECIFIED.);
#239=B_SPLINE_CURVE_WITH_KNOTS('',3,(#11083,#11084,#11085,#11086,#11087,
#11088,#11089,#11090,#11091,#11092,#11093,#11094,#11095,#11096,#11097,#11098,
#11099,#11100,#11101,#11102,#11103,#11104,#11105,#11106,#11107,#11108,#11109,
#11110),.UNSPECIFIED.,.F.,.F.,(4,3,3,3,3,3,3,3,3,4),(-0.152284734818265,
-0.128510300097745,-0.115243636037359,-0.0914764658269932,-0.0870316758632336,
-0.078197793898112,-0.0542955901223581,-0.0391042908842167,-0.0153462458625635,
0.),.UNSPECIFIED.);
#240=B_SPLINE_CURVE_WITH_KNOTS('',3,(#11111,#11112,#11113,#11114,#11115,
#11116),.UNSPECIFIED.,.F.,.F.,(4,2,4),(-0.606273164239037,-0.303762187833104,
-0.000133245189939568),.UNSPECIFIED.);
#241=B_SPLINE_CURVE_WITH_KNOTS('',3,(#11133,#11134,#11135,#11136),
 .UNSPECIFIED.,.F.,.F.,(4,4),(-12.1227852464729,-8.92068531110742),
 .UNSPECIFIED.);
#242=B_SPLINE_CURVE_WITH_KNOTS('',3,(#11177,#11178,#11179,#11180),
 .UNSPECIFIED.,.F.,.F.,(4,4),(-4.26560157995882,-1.06350164459338),
 .UNSPECIFIED.);
#243=B_SPLINE_CURVE_WITH_KNOTS('',3,(#11199,#11200,#11201,#11202,#11203,
#11204),.UNSPECIFIED.,.F.,.F.,(4,2,4),(-0.607545900263938,-0.303784727094449,
-0.00134539382494125),.UNSPECIFIED.);
#244=B_SPLINE_CURVE_WITH_KNOTS('',3,(#11206,#11207,#11208,#11209,#11210,
#11211,#11212,#11213,#11214,#11215,#11216,#11217,#11218,#11219,#11220,#11221,
#11222,#11223,#11224,#11225,#11226,#11227,#11228,#11229,#11230,#11231,#11232,
#11233),.UNSPECIFIED.,.F.,.F.,(4,3,3,3,3,3,3,3,3,4),(-0.152214473108837,
-0.128485298747135,-0.115164309990209,-0.0912534321321267,-0.0781163092888813,
-0.0652482412471129,-0.0414606388666645,-0.0390548598067502,-0.0152611452145655,
0.),.UNSPECIFIED.);
#245=B_SPLINE_CURVE_WITH_KNOTS('',3,(#11237,#11238,#11239,#11240,#11241,
#11242,#11243,#11244,#11245,#11246,#11247,#11248,#11249,#11250,#11251,#11252,
#11253,#11254,#11255,#11256,#11257,#11258,#11259,#11260,#11261,#11262,#11263,
#11264),.UNSPECIFIED.,.F.,.F.,(4,3,3,3,3,3,3,3,3,4),(-0.152216110966007,
-0.128438825687404,-0.115191384846861,-0.0914281188167518,-0.0869870566155827,
-0.0781642271790374,-0.0542662950786889,-0.0390848818783988,-0.0153309789665,
0.),.UNSPECIFIED.);
#246=B_SPLINE_CURVE_WITH_KNOTS('',3,(#11265,#11266,#11267,#11268,#11269,
#11270),.UNSPECIFIED.,.F.,.F.,(4,2,4),(-0.606227037063105,-0.303784766192107,
-2.65251918123988E-5),.UNSPECIFIED.);
#247=B_SPLINE_CURVE_WITH_KNOTS('',3,(#11288,#11289,#11290,#11291),
 .UNSPECIFIED.,.F.,.F.,(4,4),(0.0107208554739345,0.617725317592517),
 .UNSPECIFIED.);
#248=B_SPLINE_CURVE_WITH_KNOTS('',3,(#11292,#11293,#11294,#11295),
 .UNSPECIFIED.,.F.,.F.,(4,4),(-12.893479658151,-12.3228618033436),
 .UNSPECIFIED.);
#249=B_SPLINE_CURVE_WITH_KNOTS('',3,(#11318,#11319,#11320,#11321),
 .UNSPECIFIED.,.F.,.F.,(4,4),(12.3251818525939,12.893479658151),
 .UNSPECIFIED.);
#250=B_SPLINE_CURVE_WITH_KNOTS('',3,(#11325,#11326,#11327,#11328),
 .UNSPECIFIED.,.F.,.F.,(4,4),(0.292807233425235,0.861105038472338),
 .UNSPECIFIED.);
#251=B_SPLINE_CURVE_WITH_KNOTS('',3,(#11346,#11347,#11348,#11349),
 .UNSPECIFIED.,.F.,.F.,(4,4),(-0.863425087722636,-0.29280723291527),
 .UNSPECIFIED.);
#252=B_SPLINE_CURVE_WITH_KNOTS('',3,(#11350,#11351,#11352,#11353),
 .UNSPECIFIED.,.F.,.F.,(4,4),(-0.617725317592517,-0.0107208554739345),
 .UNSPECIFIED.);
#253=B_SPLINE_CURVE_WITH_KNOTS('',3,(#11437,#11438,#11439,#11440),
 .UNSPECIFIED.,.F.,.F.,(4,4),(0.00878563933291533,0.615688454110788),
 .UNSPECIFIED.);
#254=B_SPLINE_CURVE_WITH_KNOTS('',3,(#11465,#11466,#11467,#11468),
 .UNSPECIFIED.,.F.,.F.,(4,4),(-0.615688454110787,-0.00878563933291527),
 .UNSPECIFIED.);
#255=B_SPLINE_CURVE_WITH_KNOTS('',3,(#11554,#11555,#11556,#11557),
 .UNSPECIFIED.,.F.,.F.,(4,4),(-9.62771529167128E-17,0.617725317592517),
 .UNSPECIFIED.);
#256=B_SPLINE_CURVE_WITH_KNOTS('',3,(#11558,#11559,#11560,#11561),
 .UNSPECIFIED.,.F.,.F.,(4,4),(-0.617725317592517,-0.000337488966422091),
 .UNSPECIFIED.);
#257=B_SPLINE_CURVE_WITH_KNOTS('',3,(#11597,#11598,#11599,#11600,#11601),
 .UNSPECIFIED.,.F.,.F.,(4,1,4),(-12.893479658151,-5.71764434212835,-0.335767855111383),
 .UNSPECIFIED.);
#258=B_SPLINE_CURVE_WITH_KNOTS('',3,(#11602,#11603,#11604,#11605,#11606),
 .UNSPECIFIED.,.F.,.F.,(4,1,4),(0.335767855111383,5.71764434212835,12.893479658151),
 .UNSPECIFIED.);
#259=B_SPLINE_CURVE_WITH_KNOTS('',3,(#11631,#11632,#11633,#11634),
 .UNSPECIFIED.,.F.,.F.,(4,4),(-0.00171041937131743,0.615688454110788),
 .UNSPECIFIED.);
#260=B_SPLINE_CURVE_WITH_KNOTS('',3,(#11635,#11636,#11637,#11638),
 .UNSPECIFIED.,.F.,.F.,(4,4),(-0.615688454110788,-3.98826847727851E-7),
 .UNSPECIFIED.);
#261=B_SPLINE_CURVE_WITH_KNOTS('',3,(#11663,#11664,#11665,#11666),
 .UNSPECIFIED.,.F.,.F.,(4,4),(3.98826847219577E-7,0.615688454110787),
 .UNSPECIFIED.);
#262=B_SPLINE_CURVE_WITH_KNOTS('',3,(#11667,#11668,#11669,#11670),
 .UNSPECIFIED.,.F.,.F.,(4,4),(-0.615688454110787,0.0017104193713176),
 .UNSPECIFIED.);
#263=B_SPLINE_CURVE_WITH_KNOTS('',3,(#11696,#11697,#11698,#11699,#11700),
 .UNSPECIFIED.,.F.,.F.,(4,1,4),(-12.8505190359549,-7.4686425489379,-0.29280723291527),
 .UNSPECIFIED.);
#264=B_SPLINE_CURVE_WITH_KNOTS('',3,(#11701,#11702,#11703,#11704,#11705),
 .UNSPECIFIED.,.F.,.F.,(4,1,4),(0.292807233425236,7.4686425489379,12.8505190359549),
 .UNSPECIFIED.);
#265=B_SPLINE_CURVE_WITH_KNOTS('',3,(#11726,#11727,#11728,#11729),
 .UNSPECIFIED.,.F.,.F.,(4,4),(0.000337488966421928,0.617725317592517),
 .UNSPECIFIED.);
#266=B_SPLINE_CURVE_WITH_KNOTS('',3,(#11730,#11731,#11732,#11733),
 .UNSPECIFIED.,.F.,.F.,(4,4),(-0.617725317592517,8.06646416329215E-17),
 .UNSPECIFIED.);
#549=SHAPE_REPRESENTATION_RELATIONSHIP('SRR','None',#19669,#559);
#559=ADVANCED_BREP_SHAPE_REPRESENTATION('',(#579),#19612);
#569=STYLED_ITEM('',(#19731),#579);
#579=MANIFOLD_SOLID_BREP('Body1',#7107);
#608=FACE_BOUND('',#1321,.T.);
#609=FACE_BOUND('',#1322,.T.);
#610=FACE_BOUND('',#1323,.T.);
#611=FACE_BOUND('',#1330,.T.);
#612=FACE_BOUND('',#1333,.T.);
#613=FACE_BOUND('',#1344,.T.);
#614=FACE_BOUND('',#1346,.T.);
#615=FACE_BOUND('',#1358,.T.);
#616=FACE_BOUND('',#1367,.T.);
#617=FACE_BOUND('',#1368,.T.);
#618=FACE_BOUND('',#1369,.T.);
#619=FACE_BOUND('',#1418,.T.);
#620=FACE_BOUND('',#1419,.T.);
#621=FACE_BOUND('',#1420,.T.);
#622=FACE_BOUND('',#1421,.T.);
#623=FACE_BOUND('',#1422,.T.);
#624=FACE_BOUND('',#1423,.T.);
#707=PLANE('',#7374);
#708=PLANE('',#7391);
#709=PLANE('',#7396);
#710=PLANE('',#7402);
#711=PLANE('',#7403);
#712=PLANE('',#7404);
#713=PLANE('',#7405);
#714=PLANE('',#7406);
#715=PLANE('',#7407);
#716=PLANE('',#7408);
#717=PLANE('',#7409);
#718=PLANE('',#7411);
#719=PLANE('',#7413);
#720=PLANE('',#7414);
#721=PLANE('',#7415);
#722=PLANE('',#7416);
#723=PLANE('',#7417);
#724=PLANE('',#7418);
#725=PLANE('',#7419);
#726=PLANE('',#7420);
#727=PLANE('',#7421);
#728=PLANE('',#7422);
#729=PLANE('',#7423);
#730=PLANE('',#7427);
#731=PLANE('',#7429);
#732=PLANE('',#7430);
#733=PLANE('',#7431);
#734=PLANE('',#7432);
#735=PLANE('',#7433);
#736=PLANE('',#7434);
#737=PLANE('',#7436);
#738=PLANE('',#7453);
#739=PLANE('',#7472);
#740=PLANE('',#7473);
#741=PLANE('',#7474);
#898=FACE_OUTER_BOUND('',#1320,.T.);
#899=FACE_OUTER_BOUND('',#1324,.T.);
#900=FACE_OUTER_BOUND('',#1325,.T.);
#901=FACE_OUTER_BOUND('',#1326,.T.);
#902=FACE_OUTER_BOUND('',#1327,.T.);
#903=FACE_OUTER_BOUND('',#1328,.T.);
#904=FACE_OUTER_BOUND('',#1329,.T.);
#905=FACE_OUTER_BOUND('',#1331,.T.);
#906=FACE_OUTER_BOUND('',#1332,.T.);
#907=FACE_OUTER_BOUND('',#1334,.T.);
#908=FACE_OUTER_BOUND('',#1335,.T.);
#909=FACE_OUTER_BOUND('',#1336,.T.);
#910=FACE_OUTER_BOUND('',#1337,.T.);
#911=FACE_OUTER_BOUND('',#1338,.T.);
#912=FACE_OUTER_BOUND('',#1339,.T.);
#913=FACE_OUTER_BOUND('',#1340,.T.);
#914=FACE_OUTER_BOUND('',#1341,.T.);
#915=FACE_OUTER_BOUND('',#1342,.T.);
#916=FACE_OUTER_BOUND('',#1343,.T.);
#917=FACE_OUTER_BOUND('',#1345,.T.);
#918=FACE_OUTER_BOUND('',#1347,.T.);
#919=FACE_OUTER_BOUND('',#1348,.T.);
#920=FACE_OUTER_BOUND('',#1349,.T.);
#921=FACE_OUTER_BOUND('',#1350,.T.);
#922=FACE_OUTER_BOUND('',#1351,.T.);
#923=FACE_OUTER_BOUND('',#1352,.T.);
#924=FACE_OUTER_BOUND('',#1353,.T.);
#925=FACE_OUTER_BOUND('',#1354,.T.);
#926=FACE_OUTER_BOUND('',#1355,.T.);
#927=FACE_OUTER_BOUND('',#1356,.T.);
#928=FACE_OUTER_BOUND('',#1357,.T.);
#929=FACE_OUTER_BOUND('',#1359,.T.);
#930=FACE_OUTER_BOUND('',#1360,.T.);
#931=FACE_OUTER_BOUND('',#1361,.T.);
#932=FACE_OUTER_BOUND('',#1362,.T.);
#933=FACE_OUTER_BOUND('',#1363,.T.);
#934=FACE_OUTER_BOUND('',#1364,.T.);
#935=FACE_OUTER_BOUND('',#1365,.T.);
#936=FACE_OUTER_BOUND('',#1366,.T.);
#937=FACE_OUTER_BOUND('',#1370,.T.);
#938=FACE_OUTER_BOUND('',#1371,.T.);
#939=FACE_OUTER_BOUND('',#1372,.T.);
#940=FACE_OUTER_BOUND('',#1373,.T.);
#941=FACE_OUTER_BOUND('',#1374,.T.);
#942=FACE_OUTER_BOUND('',#1375,.T.);
#943=FACE_OUTER_BOUND('',#1376,.T.);
#944=FACE_OUTER_BOUND('',#1377,.T.);
#945=FACE_OUTER_BOUND('',#1378,.T.);
#946=FACE_OUTER_BOUND('',#1379,.T.);
#947=FACE_OUTER_BOUND('',#1380,.T.);
#948=FACE_OUTER_BOUND('',#1381,.T.);
#949=FACE_OUTER_BOUND('',#1382,.T.);
#950=FACE_OUTER_BOUND('',#1383,.T.);
#951=FACE_OUTER_BOUND('',#1384,.T.);
#952=FACE_OUTER_BOUND('',#1385,.T.);
#953=FACE_OUTER_BOUND('',#1386,.T.);
#954=FACE_OUTER_BOUND('',#1387,.T.);
#955=FACE_OUTER_BOUND('',#1388,.T.);
#956=FACE_OUTER_BOUND('',#1389,.T.);
#957=FACE_OUTER_BOUND('',#1390,.T.);
#958=FACE_OUTER_BOUND('',#1391,.T.);
#959=FACE_OUTER_BOUND('',#1392,.T.);
#960=FACE_OUTER_BOUND('',#1393,.T.);
#961=FACE_OUTER_BOUND('',#1394,.T.);
#962=FACE_OUTER_BOUND('',#1395,.T.);
#963=FACE_OUTER_BOUND('',#1396,.T.);
#964=FACE_OUTER_BOUND('',#1397,.T.);
#965=FACE_OUTER_BOUND('',#1398,.T.);
#966=FACE_OUTER_BOUND('',#1399,.T.);
#967=FACE_OUTER_BOUND('',#1400,.T.);
#968=FACE_OUTER_BOUND('',#1401,.T.);
#969=FACE_OUTER_BOUND('',#1402,.T.);
#970=FACE_OUTER_BOUND('',#1403,.T.);
#971=FACE_OUTER_BOUND('',#1404,.T.);
#972=FACE_OUTER_BOUND('',#1405,.T.);
#973=FACE_OUTER_BOUND('',#1406,.T.);
#974=FACE_OUTER_BOUND('',#1407,.T.);
#975=FACE_OUTER_BOUND('',#1408,.T.);
#976=FACE_OUTER_BOUND('',#1409,.T.);
#977=FACE_OUTER_BOUND('',#1410,.T.);
#978=FACE_OUTER_BOUND('',#1411,.T.);
#979=FACE_OUTER_BOUND('',#1412,.T.);
#980=FACE_OUTER_BOUND('',#1413,.T.);
#981=FACE_OUTER_BOUND('',#1414,.T.);
#982=FACE_OUTER_BOUND('',#1415,.T.);
#983=FACE_OUTER_BOUND('',#1416,.T.);
#984=FACE_OUTER_BOUND('',#1417,.T.);
#985=FACE_OUTER_BOUND('',#1424,.T.);
#986=FACE_OUTER_BOUND('',#1425,.T.);
#1320=EDGE_LOOP('',(#4890,#4891,#4892,#4893,#4894,#4895,#4896,#4897));
#1321=EDGE_LOOP('',(#4898));
#1322=EDGE_LOOP('',(#4899));
#1323=EDGE_LOOP('',(#4900));
#1324=EDGE_LOOP('',(#4901,#4902,#4903,#4904));
#1325=EDGE_LOOP('',(#4905,#4906,#4907,#4908));
#1326=EDGE_LOOP('',(#4909,#4910,#4911,#4912));
#1327=EDGE_LOOP('',(#4913,#4914,#4915,#4916));
#1328=EDGE_LOOP('',(#4917,#4918,#4919,#4920));
#1329=EDGE_LOOP('',(#4921));
#1330=EDGE_LOOP('',(#4922));
#1331=EDGE_LOOP('',(#4923,#4924,#4925,#4926));
#1332=EDGE_LOOP('',(#4927));
#1333=EDGE_LOOP('',(#4928));
#1334=EDGE_LOOP('',(#4929,#4930,#4931,#4932));
#1335=EDGE_LOOP('',(#4933,#4934,#4935,#4936));
#1336=EDGE_LOOP('',(#4937,#4938,#4939,#4940));
#1337=EDGE_LOOP('',(#4941,#4942,#4943,#4944));
#1338=EDGE_LOOP('',(#4945,#4946,#4947,#4948));
#1339=EDGE_LOOP('',(#4949,#4950,#4951,#4952));
#1340=EDGE_LOOP('',(#4953,#4954,#4955,#4956));
#1341=EDGE_LOOP('',(#4957,#4958,#4959,#4960));
#1342=EDGE_LOOP('',(#4961,#4962,#4963,#4964));
#1343=EDGE_LOOP('',(#4965));
#1344=EDGE_LOOP('',(#4966));
#1345=EDGE_LOOP('',(#4967));
#1346=EDGE_LOOP('',(#4968));
#1347=EDGE_LOOP('',(#4969,#4970,#4971,#4972));
#1348=EDGE_LOOP('',(#4973,#4974,#4975,#4976));
#1349=EDGE_LOOP('',(#4977,#4978,#4979,#4980));
#1350=EDGE_LOOP('',(#4981,#4982,#4983,#4984));
#1351=EDGE_LOOP('',(#4985,#4986,#4987,#4988));
#1352=EDGE_LOOP('',(#4989,#4990,#4991,#4992,#4993,#4994));
#1353=EDGE_LOOP('',(#4995,#4996,#4997,#4998,#4999,#5000,#5001,#5002,#5003,
#5004));
#1354=EDGE_LOOP('',(#5005,#5006,#5007,#5008,#5009,#5010,#5011,#5012,#5013,
#5014));
#1355=EDGE_LOOP('',(#5015,#5016,#5017,#5018,#5019,#5020,#5021,#5022,#5023,
#5024));
#1356=EDGE_LOOP('',(#5025,#5026,#5027,#5028,#5029,#5030,#5031,#5032));
#1357=EDGE_LOOP('',(#5033,#5034,#5035,#5036,#5037,#5038,#5039,#5040,#5041,
#5042,#5043,#5044,#5045,#5046,#5047,#5048,#5049,#5050,#5051,#5052,#5053,
#5054,#5055,#5056,#5057,#5058,#5059,#5060,#5061,#5062,#5063,#5064,#5065,
#5066,#5067,#5068,#5069,#5070,#5071,#5072,#5073,#5074));
#1358=EDGE_LOOP('',(#5075,#5076,#5077,#5078,#5079,#5080));
#1359=EDGE_LOOP('',(#5081,#5082,#5083,#5084));
#1360=EDGE_LOOP('',(#5085,#5086,#5087,#5088));
#1361=EDGE_LOOP('',(#5089,#5090,#5091,#5092,#5093,#5094));
#1362=EDGE_LOOP('',(#5095,#5096,#5097,#5098));
#1363=EDGE_LOOP('',(#5099,#5100,#5101,#5102));
#1364=EDGE_LOOP('',(#5103,#5104,#5105,#5106));
#1365=EDGE_LOOP('',(#5107,#5108,#5109,#5110));
#1366=EDGE_LOOP('',(#5111,#5112,#5113,#5114));
#1367=EDGE_LOOP('',(#5115));
#1368=EDGE_LOOP('',(#5116));
#1369=EDGE_LOOP('',(#5117));
#1370=EDGE_LOOP('',(#5118,#5119,#5120,#5121));
#1371=EDGE_LOOP('',(#5122,#5123,#5124,#5125));
#1372=EDGE_LOOP('',(#5126,#5127,#5128,#5129));
#1373=EDGE_LOOP('',(#5130,#5131,#5132,#5133));
#1374=EDGE_LOOP('',(#5134,#5135,#5136,#5137,#5138,#5139,#5140,#5141,#5142,
#5143));
#1375=EDGE_LOOP('',(#5144,#5145,#5146,#5147));
#1376=EDGE_LOOP('',(#5148,#5149,#5150,#5151));
#1377=EDGE_LOOP('',(#5152,#5153,#5154,#5155));
#1378=EDGE_LOOP('',(#5156,#5157,#5158,#5159));
#1379=EDGE_LOOP('',(#5160,#5161,#5162,#5163));
#1380=EDGE_LOOP('',(#5164,#5165,#5166,#5167,#5168,#5169,#5170,#5171,#5172,
#5173));
#1381=EDGE_LOOP('',(#5174,#5175,#5176,#5177));
#1382=EDGE_LOOP('',(#5178,#5179,#5180,#5181,#5182,#5183));
#1383=EDGE_LOOP('',(#5184,#5185,#5186,#5187,#5188,#5189));
#1384=EDGE_LOOP('',(#5190,#5191,#5192,#5193));
#1385=EDGE_LOOP('',(#5194,#5195,#5196,#5197,#5198,#5199,#5200,#5201,#5202,
#5203));
#1386=EDGE_LOOP('',(#5204,#5205,#5206,#5207));
#1387=EDGE_LOOP('',(#5208,#5209,#5210,#5211));
#1388=EDGE_LOOP('',(#5212,#5213,#5214,#5215));
#1389=EDGE_LOOP('',(#5216,#5217,#5218,#5219));
#1390=EDGE_LOOP('',(#5220,#5221,#5222,#5223));
#1391=EDGE_LOOP('',(#5224,#5225,#5226));
#1392=EDGE_LOOP('',(#5227,#5228,#5229));
#1393=EDGE_LOOP('',(#5230,#5231,#5232));
#1394=EDGE_LOOP('',(#5233,#5234,#5235,#5236));
#1395=EDGE_LOOP('',(#5237,#5238,#5239,#5240));
#1396=EDGE_LOOP('',(#5241,#5242,#5243));
#1397=EDGE_LOOP('',(#5244,#5245,#5246,#5247));
#1398=EDGE_LOOP('',(#5248,#5249,#5250,#5251));
#1399=EDGE_LOOP('',(#5252,#5253,#5254,#5255));
#1400=EDGE_LOOP('',(#5256,#5257,#5258,#5259));
#1401=EDGE_LOOP('',(#5260,#5261,#5262,#5263));
#1402=EDGE_LOOP('',(#5264,#5265,#5266,#5267));
#1403=EDGE_LOOP('',(#5268,#5269,#5270));
#1404=EDGE_LOOP('',(#5271,#5272,#5273));
#1405=EDGE_LOOP('',(#5274,#5275,#5276));
#1406=EDGE_LOOP('',(#5277,#5278,#5279,#5280));
#1407=EDGE_LOOP('',(#5281,#5282,#5283,#5284));
#1408=EDGE_LOOP('',(#5285,#5286,#5287));
#1409=EDGE_LOOP('',(#5288,#5289,#5290,#5291));
#1410=EDGE_LOOP('',(#5292,#5293,#5294,#5295));
#1411=EDGE_LOOP('',(#5296,#5297,#5298,#5299));
#1412=EDGE_LOOP('',(#5300,#5301,#5302,#5303));
#1413=EDGE_LOOP('',(#5304,#5305,#5306,#5307));
#1414=EDGE_LOOP('',(#5308,#5309,#5310,#5311));
#1415=EDGE_LOOP('',(#5312,#5313,#5314,#5315));
#1416=EDGE_LOOP('',(#5316,#5317,#5318,#5319,#5320,#5321,#5322,#5323));
#1417=EDGE_LOOP('',(#5324,#5325,#5326,#5327));
#1418=EDGE_LOOP('',(#5328));
#1419=EDGE_LOOP('',(#5329));
#1420=EDGE_LOOP('',(#5330));
#1421=EDGE_LOOP('',(#5331));
#1422=EDGE_LOOP('',(#5332));
#1423=EDGE_LOOP('',(#5333));
#1424=EDGE_LOOP('',(#5334,#5335,#5336,#5337));
#1425=EDGE_LOOP('',(#5338,#5339,#5340,#5341));
#1825=LINE('',#9730,#2284);
#1826=LINE('',#9762,#2285);
#1827=LINE('',#9797,#2286);
#1828=LINE('',#9802,#2287);
#1829=LINE('',#9806,#2288);
#1830=LINE('',#9811,#2289);
#1831=LINE('',#9817,#2290);
#1832=LINE('',#9826,#2291);
#1833=LINE('',#9833,#2292);
#1834=LINE('',#9837,#2293);
#1835=LINE('',#9842,#2294);
#1836=LINE('',#9844,#2295);
#1837=LINE('',#9846,#2296);
#1838=LINE('',#9847,#2297);
#1839=LINE('',#9851,#2298);
#1840=LINE('',#9853,#2299);
#1841=LINE('',#9855,#2300);
#1842=LINE('',#9856,#2301);
#1843=LINE('',#9860,#2302);
#1844=LINE('',#9862,#2303);
#1845=LINE('',#9864,#2304);
#1846=LINE('',#9865,#2305);
#1847=LINE('',#9869,#2306);
#1848=LINE('',#9871,#2307);
#1849=LINE('',#9873,#2308);
#1850=LINE('',#9874,#2309);
#1851=LINE('',#9878,#2310);
#1852=LINE('',#9880,#2311);
#1853=LINE('',#9882,#2312);
#1854=LINE('',#9883,#2313);
#1855=LINE('',#9887,#2314);
#1856=LINE('',#9889,#2315);
#1857=LINE('',#9891,#2316);
#1858=LINE('',#9892,#2317);
#1859=LINE('',#9896,#2318);
#1860=LINE('',#9898,#2319);
#1861=LINE('',#9900,#2320);
#1862=LINE('',#9901,#2321);
#1863=LINE('',#9909,#2322);
#1864=LINE('',#9910,#2323);
#1865=LINE('',#9912,#2324);
#1866=LINE('',#9913,#2325);
#1867=LINE('',#9915,#2326);
#1868=LINE('',#9916,#2327);
#1869=LINE('',#9919,#2328);
#1870=LINE('',#9921,#2329);
#1871=LINE('',#9922,#2330);
#1872=LINE('',#9925,#2331);
#1873=LINE('',#9927,#2332);
#1874=LINE('',#9928,#2333);
#1875=LINE('',#9932,#2334);
#1876=LINE('',#9970,#2335);
#1877=LINE('',#10008,#2336);
#1878=LINE('',#10046,#2337);
#1879=LINE('',#10083,#2338);
#1880=LINE('',#10086,#2339);
#1881=LINE('',#10124,#2340);
#1882=LINE('',#10161,#2341);
#1883=LINE('',#10164,#2342);
#1884=LINE('',#10236,#2343);
#1885=LINE('',#10239,#2344);
#1886=LINE('',#10246,#2345);
#1887=LINE('',#10252,#2346);
#1888=LINE('',#10263,#2347);
#1889=LINE('',#10275,#2348);
#1890=LINE('',#10281,#2349);
#1891=LINE('',#10316,#2350);
#1892=LINE('',#10405,#2351);
#1893=LINE('',#10493,#2352);
#1894=LINE('',#10528,#2353);
#1895=LINE('',#10534,#2354);
#1896=LINE('',#10546,#2355);
#1897=LINE('',#10589,#2356);
#1898=LINE('',#10630,#2357);
#1899=LINE('',#10634,#2358);
#1900=LINE('',#10636,#2359);
#1901=LINE('',#10682,#2360);
#1902=LINE('',#10817,#2361);
#1903=LINE('',#10921,#2362);
#1904=LINE('',#11235,#2363);
#1905=LINE('',#11324,#2364);
#1906=LINE('',#11412,#2365);
#1907=LINE('',#11532,#2366);
#1908=LINE('',#11533,#2367);
#1909=LINE('',#11570,#2368);
#1910=LINE('',#11571,#2369);
#2284=VECTOR('',#8198,1.);
#2285=VECTOR('',#8199,1.);
#2286=VECTOR('',#8210,0.15);
#2287=VECTOR('',#8217,0.15);
#2288=VECTOR('',#8222,0.15);
#2289=VECTOR('',#8227,0.15);
#2290=VECTOR('',#8234,0.3);
#2291=VECTOR('',#8245,0.3);
#2292=VECTOR('',#8254,0.17);
#2293=VECTOR('',#8259,0.17);
#2294=VECTOR('',#8264,1.);
#2295=VECTOR('',#8265,1.);
#2296=VECTOR('',#8266,1.);
#2297=VECTOR('',#8267,1.);
#2298=VECTOR('',#8270,1.);
#2299=VECTOR('',#8271,1.);
#2300=VECTOR('',#8272,1.);
#2301=VECTOR('',#8273,1.);
#2302=VECTOR('',#8276,1.);
#2303=VECTOR('',#8277,1.);
#2304=VECTOR('',#8278,1.);
#2305=VECTOR('',#8279,1.);
#2306=VECTOR('',#8282,1.);
#2307=VECTOR('',#8283,1.);
#2308=VECTOR('',#8284,1.);
#2309=VECTOR('',#8285,1.);
#2310=VECTOR('',#8288,1.);
#2311=VECTOR('',#8289,1.);
#2312=VECTOR('',#8290,1.);
#2313=VECTOR('',#8291,1.);
#2314=VECTOR('',#8294,1.);
#2315=VECTOR('',#8295,1.);
#2316=VECTOR('',#8296,1.);
#2317=VECTOR('',#8297,1.);
#2318=VECTOR('',#8300,1.);
#2319=VECTOR('',#8301,1.);
#2320=VECTOR('',#8302,1.);
#2321=VECTOR('',#8303,1.);
#2322=VECTOR('',#8314,1.);
#2323=VECTOR('',#8315,1.);
#2324=VECTOR('',#8318,1.);
#2325=VECTOR('',#8319,1.);
#2326=VECTOR('',#8322,1.);
#2327=VECTOR('',#8323,1.);
#2328=VECTOR('',#8326,1.);
#2329=VECTOR('',#8327,1.);
#2330=VECTOR('',#8328,1.);
#2331=VECTOR('',#8331,1.);
#2332=VECTOR('',#8332,1.);
#2333=VECTOR('',#8333,1.);
#2334=VECTOR('',#8336,1.);
#2335=VECTOR('',#8337,1.);
#2336=VECTOR('',#8340,1.);
#2337=VECTOR('',#8341,1.);
#2338=VECTOR('',#8342,1.);
#2339=VECTOR('',#8345,1.);
#2340=VECTOR('',#8346,1.);
#2341=VECTOR('',#8347,1.);
#2342=VECTOR('',#8350,1.);
#2343=VECTOR('',#8351,1.);
#2344=VECTOR('',#8354,1.);
#2345=VECTOR('',#8355,1.);
#2346=VECTOR('',#8356,1.);
#2347=VECTOR('',#8359,1.);
#2348=VECTOR('',#8360,1.);
#2349=VECTOR('',#8361,1.);
#2350=VECTOR('',#8362,1.);
#2351=VECTOR('',#8363,1.);
#2352=VECTOR('',#8364,1.);
#2353=VECTOR('',#8365,1.);
#2354=VECTOR('',#8366,1.);
#2355=VECTOR('',#8367,1.);
#2356=VECTOR('',#8368,1.);
#2357=VECTOR('',#8369,1.);
#2358=VECTOR('',#8374,0.4);
#2359=VECTOR('',#8377,0.4);
#2360=VECTOR('',#8380,1.);
#2361=VECTOR('',#8387,1.);
#2362=VECTOR('',#8390,1.);
#2363=VECTOR('',#8397,1.);
#2364=VECTOR('',#8402,1.);
#2365=VECTOR('',#8435,1.);
#2366=VECTOR('',#8464,1.);
#2367=VECTOR('',#8465,1.);
#2368=VECTOR('',#8476,1.);
#2369=VECTOR('',#8477,1.);
#2682=CIRCLE('',#7375,0.15);
#2683=CIRCLE('',#7376,0.15);
#2684=CIRCLE('',#7377,0.4);
#2685=CIRCLE('',#7379,0.15);
#2686=CIRCLE('',#7380,0.15);
#2687=CIRCLE('',#7382,0.15);
#2688=CIRCLE('',#7384,0.15);
#2689=CIRCLE('',#7386,0.15);
#2690=CIRCLE('',#7387,0.15);
#2691=CIRCLE('',#7389,0.3);
#2692=CIRCLE('',#7390,0.3);
#2693=CIRCLE('',#7392,0.17);
#2694=CIRCLE('',#7394,0.3);
#2695=CIRCLE('',#7395,0.3);
#2696=CIRCLE('',#7397,0.17);
#2697=CIRCLE('',#7399,0.17);
#2698=CIRCLE('',#7401,0.17);
#2699=CIRCLE('',#7410,0.4);
#2700=CIRCLE('',#7412,0.4);
#2701=CIRCLE('',#7425,0.4);
#2702=CIRCLE('',#7428,0.1);
#2703=CIRCLE('',#7435,0.0999999999999999);
#2704=CIRCLE('',#7437,0.0999999999999999);
#2705=CIRCLE('',#7439,0.0999999999999999);
#2706=CIRCLE('',#7440,0.1);
#2707=CIRCLE('',#7442,0.0999999999999998);
#2708=CIRCLE('',#7443,0.0999999999999998);
#2709=CIRCLE('',#7444,0.0999999999999997);
#2710=CIRCLE('',#7446,0.0999999999999998);
#2711=CIRCLE('',#7447,0.0999999999999998);
#2712=CIRCLE('',#7450,0.0999999999999999);
#2713=CIRCLE('',#7451,0.1);
#2714=CIRCLE('',#7455,0.3);
#2715=CIRCLE('',#7456,0.3);
#2716=CIRCLE('',#7457,0.3);
#2717=CIRCLE('',#7459,0.3);
#2718=CIRCLE('',#7460,0.3);
#2719=CIRCLE('',#7461,0.3);
#2720=CIRCLE('',#7463,0.3);
#2721=CIRCLE('',#7464,0.3);
#2722=CIRCLE('',#7465,0.3);
#2723=CIRCLE('',#7468,0.3);
#2724=CIRCLE('',#7469,0.3);
#2725=CIRCLE('',#7470,0.3);
#2937=VERTEX_POINT('',#9723);
#2938=VERTEX_POINT('',#9724);
#2939=VERTEX_POINT('',#9729);
#2940=VERTEX_POINT('',#9731);
#2941=VERTEX_POINT('',#9736);
#2942=VERTEX_POINT('',#9756);
#2943=VERTEX_POINT('',#9761);
#2944=VERTEX_POINT('',#9763);
#2945=VERTEX_POINT('',#9787);
#2946=VERTEX_POINT('',#9789);
#2947=VERTEX_POINT('',#9791);
#2948=VERTEX_POINT('',#9794);
#2949=VERTEX_POINT('',#9796);
#2950=VERTEX_POINT('',#9800);
#2951=VERTEX_POINT('',#9804);
#2952=VERTEX_POINT('',#9808);
#2953=VERTEX_POINT('',#9810);
#2954=VERTEX_POINT('',#9814);
#2955=VERTEX_POINT('',#9816);
#2956=VERTEX_POINT('',#9820);
#2957=VERTEX_POINT('',#9823);
#2958=VERTEX_POINT('',#9825);
#2959=VERTEX_POINT('',#9829);
#2960=VERTEX_POINT('',#9832);
#2961=VERTEX_POINT('',#9836);
#2962=VERTEX_POINT('',#9840);
#2963=VERTEX_POINT('',#9841);
#2964=VERTEX_POINT('',#9843);
#2965=VERTEX_POINT('',#9845);
#2966=VERTEX_POINT('',#9849);
#2967=VERTEX_POINT('',#9850);
#2968=VERTEX_POINT('',#9852);
#2969=VERTEX_POINT('',#9854);
#2970=VERTEX_POINT('',#9858);
#2971=VERTEX_POINT('',#9859);
#2972=VERTEX_POINT('',#9861);
#2973=VERTEX_POINT('',#9863);
#2974=VERTEX_POINT('',#9867);
#2975=VERTEX_POINT('',#9868);
#2976=VERTEX_POINT('',#9870);
#2977=VERTEX_POINT('',#9872);
#2978=VERTEX_POINT('',#9876);
#2979=VERTEX_POINT('',#9877);
#2980=VERTEX_POINT('',#9879);
#2981=VERTEX_POINT('',#9881);
#2982=VERTEX_POINT('',#9885);
#2983=VERTEX_POINT('',#9886);
#2984=VERTEX_POINT('',#9888);
#2985=VERTEX_POINT('',#9890);
#2986=VERTEX_POINT('',#9894);
#2987=VERTEX_POINT('',#9895);
#2988=VERTEX_POINT('',#9897);
#2989=VERTEX_POINT('',#9899);
#2990=VERTEX_POINT('',#9903);
#2991=VERTEX_POINT('',#9906);
#2992=VERTEX_POINT('',#9918);
#2993=VERTEX_POINT('',#9920);
#2994=VERTEX_POINT('',#9924);
#2995=VERTEX_POINT('',#9926);
#2996=VERTEX_POINT('',#9930);
#2997=VERTEX_POINT('',#9931);
#2998=VERTEX_POINT('',#9933);
#2999=VERTEX_POINT('',#9940);
#3000=VERTEX_POINT('',#9969);
#3001=VERTEX_POINT('',#9971);
#3002=VERTEX_POINT('',#10007);
#3003=VERTEX_POINT('',#10009);
#3004=VERTEX_POINT('',#10016);
#3005=VERTEX_POINT('',#10045);
#3006=VERTEX_POINT('',#10047);
#3007=VERTEX_POINT('',#10076);
#3008=VERTEX_POINT('',#10085);
#3009=VERTEX_POINT('',#10087);
#3010=VERTEX_POINT('',#10094);
#3011=VERTEX_POINT('',#10123);
#3012=VERTEX_POINT('',#10125);
#3013=VERTEX_POINT('',#10154);
#3014=VERTEX_POINT('',#10163);
#3015=VERTEX_POINT('',#10165);
#3016=VERTEX_POINT('',#10200);
#3017=VERTEX_POINT('',#10229);
#3018=VERTEX_POINT('',#10238);
#3019=VERTEX_POINT('',#10240);
#3020=VERTEX_POINT('',#10245);
#3021=VERTEX_POINT('',#10247);
#3022=VERTEX_POINT('',#10262);
#3023=VERTEX_POINT('',#10274);
#3024=VERTEX_POINT('',#10280);
#3025=VERTEX_POINT('',#10282);
#3026=VERTEX_POINT('',#10315);
#3027=VERTEX_POINT('',#10317);
#3028=VERTEX_POINT('',#10355);
#3029=VERTEX_POINT('',#10360);
#3030=VERTEX_POINT('',#10404);
#3031=VERTEX_POINT('',#10406);
#3032=VERTEX_POINT('',#10450);
#3033=VERTEX_POINT('',#10455);
#3034=VERTEX_POINT('',#10494);
#3035=VERTEX_POINT('',#10523);
#3036=VERTEX_POINT('',#10529);
#3037=VERTEX_POINT('',#10535);
#3038=VERTEX_POINT('',#10547);
#3039=VERTEX_POINT('',#10548);
#3040=VERTEX_POINT('',#10553);
#3041=VERTEX_POINT('',#10588);
#3042=VERTEX_POINT('',#10590);
#3043=VERTEX_POINT('',#10625);
#3044=VERTEX_POINT('',#10632);
#3045=VERTEX_POINT('',#10638);
#3046=VERTEX_POINT('',#10645);
#3047=VERTEX_POINT('',#10652);
#3048=VERTEX_POINT('',#10681);
#3049=VERTEX_POINT('',#10747);
#3050=VERTEX_POINT('',#10800);
#3051=VERTEX_POINT('',#10812);
#3052=VERTEX_POINT('',#10874);
#3053=VERTEX_POINT('',#10884);
#3054=VERTEX_POINT('',#10891);
#3055=VERTEX_POINT('',#10920);
#3056=VERTEX_POINT('',#10922);
#3057=VERTEX_POINT('',#11047);
#3058=VERTEX_POINT('',#11082);
#3059=VERTEX_POINT('',#11198);
#3060=VERTEX_POINT('',#11205);
#3061=VERTEX_POINT('',#11234);
#3062=VERTEX_POINT('',#11236);
#3063=VERTEX_POINT('',#11287);
#3064=VERTEX_POINT('',#11316);
#3065=VERTEX_POINT('',#11323);
#3066=VERTEX_POINT('',#11345);
#3067=VERTEX_POINT('',#11380);
#3068=VERTEX_POINT('',#11408);
#3069=VERTEX_POINT('',#11511);
#3070=VERTEX_POINT('',#11512);
#3071=VERTEX_POINT('',#11514);
#3072=VERTEX_POINT('',#11518);
#3073=VERTEX_POINT('',#11519);
#3074=VERTEX_POINT('',#11521);
#3075=VERTEX_POINT('',#11525);
#3076=VERTEX_POINT('',#11526);
#3077=VERTEX_POINT('',#11528);
#3078=VERTEX_POINT('',#11563);
#3079=VERTEX_POINT('',#11564);
#3080=VERTEX_POINT('',#11566);
#3670=EDGE_CURVE('',#2937,#2938,#171,.T.);
#3671=EDGE_CURVE('',#2938,#2939,#1825,.T.);
#3672=EDGE_CURVE('',#2939,#2940,#172,.T.);
#3673=EDGE_CURVE('',#2941,#2940,#173,.T.);
#3674=EDGE_CURVE('',#2941,#2942,#174,.T.);
#3675=EDGE_CURVE('',#2942,#2943,#1826,.T.);
#3676=EDGE_CURVE('',#2943,#2944,#175,.T.);
#3677=EDGE_CURVE('',#2937,#2944,#176,.T.);
#3678=EDGE_CURVE('',#2945,#2945,#2682,.T.);
#3679=EDGE_CURVE('',#2946,#2946,#2683,.T.);
#3680=EDGE_CURVE('',#2947,#2947,#2684,.T.);
#3681=EDGE_CURVE('',#2948,#2948,#2685,.T.);
#3682=EDGE_CURVE('',#2948,#2949,#1827,.T.);
#3683=EDGE_CURVE('',#2949,#2949,#2686,.T.);
#3684=EDGE_CURVE('',#2950,#2950,#2687,.T.);
#3685=EDGE_CURVE('',#2950,#2946,#1828,.T.);
#3686=EDGE_CURVE('',#2951,#2951,#2688,.T.);
#3687=EDGE_CURVE('',#2951,#2945,#1829,.T.);
#3688=EDGE_CURVE('',#2952,#2952,#2689,.T.);
#3689=EDGE_CURVE('',#2952,#2953,#1830,.T.);
#3690=EDGE_CURVE('',#2953,#2953,#2690,.T.);
#3691=EDGE_CURVE('',#2954,#2954,#2691,.T.);
#3692=EDGE_CURVE('',#2954,#2955,#1831,.T.);
#3693=EDGE_CURVE('',#2955,#2955,#2692,.T.);
#3694=EDGE_CURVE('',#2956,#2956,#2693,.T.);
#3695=EDGE_CURVE('',#2957,#2957,#2694,.T.);
#3696=EDGE_CURVE('',#2957,#2958,#1832,.T.);
#3697=EDGE_CURVE('',#2958,#2958,#2695,.T.);
#3698=EDGE_CURVE('',#2959,#2959,#2696,.T.);
#3699=EDGE_CURVE('',#2956,#2960,#1833,.T.);
#3700=EDGE_CURVE('',#2960,#2960,#2697,.T.);
#3701=EDGE_CURVE('',#2959,#2961,#1834,.T.);
#3702=EDGE_CURVE('',#2961,#2961,#2698,.T.);
#3703=EDGE_CURVE('',#2962,#2963,#1835,.T.);
#3704=EDGE_CURVE('',#2964,#2962,#1836,.T.);
#3705=EDGE_CURVE('',#2965,#2964,#1837,.T.);
#3706=EDGE_CURVE('',#2965,#2963,#1838,.T.);
#3707=EDGE_CURVE('',#2966,#2967,#1839,.T.);
#3708=EDGE_CURVE('',#2966,#2968,#1840,.T.);
#3709=EDGE_CURVE('',#2969,#2968,#1841,.T.);
#3710=EDGE_CURVE('',#2967,#2969,#1842,.T.);
#3711=EDGE_CURVE('',#2970,#2971,#1843,.T.);
#3712=EDGE_CURVE('',#2970,#2972,#1844,.T.);
#3713=EDGE_CURVE('',#2973,#2972,#1845,.T.);
#3714=EDGE_CURVE('',#2971,#2973,#1846,.T.);
#3715=EDGE_CURVE('',#2974,#2975,#1847,.T.);
#3716=EDGE_CURVE('',#2974,#2976,#1848,.T.);
#3717=EDGE_CURVE('',#2977,#2976,#1849,.T.);
#3718=EDGE_CURVE('',#2975,#2977,#1850,.T.);
#3719=EDGE_CURVE('',#2978,#2979,#1851,.T.);
#3720=EDGE_CURVE('',#2978,#2980,#1852,.T.);
#3721=EDGE_CURVE('',#2981,#2980,#1853,.T.);
#3722=EDGE_CURVE('',#2979,#2981,#1854,.T.);
#3723=EDGE_CURVE('',#2982,#2983,#1855,.T.);
#3724=EDGE_CURVE('',#2984,#2982,#1856,.T.);
#3725=EDGE_CURVE('',#2985,#2984,#1857,.T.);
#3726=EDGE_CURVE('',#2985,#2983,#1858,.T.);
#3727=EDGE_CURVE('',#2986,#2987,#1859,.T.);
#3728=EDGE_CURVE('',#2988,#2986,#1860,.T.);
#3729=EDGE_CURVE('',#2989,#2988,#1861,.T.);
#3730=EDGE_CURVE('',#2989,#2987,#1862,.T.);
#3731=EDGE_CURVE('',#2990,#2990,#2699,.T.);
#3732=EDGE_CURVE('',#2991,#2991,#2700,.T.);
#3733=EDGE_CURVE('',#2963,#2978,#1863,.T.);
#3734=EDGE_CURVE('',#2980,#2965,#1864,.T.);
#3735=EDGE_CURVE('',#2983,#2966,#1865,.T.);
#3736=EDGE_CURVE('',#2968,#2985,#1866,.T.);
#3737=EDGE_CURVE('',#2987,#2970,#1867,.T.);
#3738=EDGE_CURVE('',#2972,#2989,#1868,.T.);
#3739=EDGE_CURVE('',#2992,#2974,#1869,.T.);
#3740=EDGE_CURVE('',#2993,#2992,#1870,.T.);
#3741=EDGE_CURVE('',#2976,#2993,#1871,.T.);
#3742=EDGE_CURVE('',#2994,#2992,#1872,.T.);
#3743=EDGE_CURVE('',#2995,#2994,#1873,.T.);
#3744=EDGE_CURVE('',#2993,#2995,#1874,.T.);
#3745=EDGE_CURVE('',#2996,#2997,#1875,.T.);
#3746=EDGE_CURVE('',#2998,#2997,#177,.T.);
#3747=EDGE_CURVE('',#2999,#2998,#178,.T.);
#3748=EDGE_CURVE('',#3000,#2999,#1876,.T.);
#3749=EDGE_CURVE('',#3001,#3000,#179,.T.);
#3750=EDGE_CURVE('',#2996,#3001,#180,.T.);
#3751=EDGE_CURVE('',#2995,#3002,#1877,.T.);
#3752=EDGE_CURVE('',#3003,#3002,#181,.T.);
#3753=EDGE_CURVE('',#3004,#3003,#182,.T.);
#3754=EDGE_CURVE('',#3005,#3004,#1878,.T.);
#3755=EDGE_CURVE('',#3006,#3005,#183,.T.);
#3756=EDGE_CURVE('',#3007,#3006,#184,.T.);
#3757=EDGE_CURVE('',#3007,#2977,#1879,.T.);
#3758=EDGE_CURVE('',#2988,#3008,#1880,.T.);
#3759=EDGE_CURVE('',#3009,#3008,#185,.T.);
#3760=EDGE_CURVE('',#3010,#3009,#186,.T.);
#3761=EDGE_CURVE('',#3011,#3010,#1881,.T.);
#3762=EDGE_CURVE('',#3012,#3011,#187,.T.);
#3763=EDGE_CURVE('',#3013,#3012,#188,.T.);
#3764=EDGE_CURVE('',#3013,#2973,#1882,.T.);
#3765=EDGE_CURVE('',#2984,#3014,#1883,.T.);
#3766=EDGE_CURVE('',#3015,#3014,#189,.T.);
#3767=EDGE_CURVE('',#2943,#3015,#190,.T.);
#3768=EDGE_CURVE('',#3016,#2942,#191,.T.);
#3769=EDGE_CURVE('',#3017,#3016,#192,.T.);
#3770=EDGE_CURVE('',#3017,#2969,#1884,.T.);
#3771=EDGE_CURVE('',#3018,#2979,#1885,.T.);
#3772=EDGE_CURVE('',#3018,#3019,#193,.T.);
#3773=EDGE_CURVE('',#3019,#3020,#1886,.T.);
#3774=EDGE_CURVE('',#3020,#3021,#194,.T.);
#3775=EDGE_CURVE('',#2962,#3021,#1887,.T.);
#3776=EDGE_CURVE('',#3007,#2997,#195,.T.);
#3777=EDGE_CURVE('',#2996,#3002,#196,.T.);
#3778=EDGE_CURVE('',#3022,#2994,#1888,.T.);
#3779=EDGE_CURVE('',#3022,#3008,#197,.T.);
#3780=EDGE_CURVE('',#3023,#2986,#1889,.T.);
#3781=EDGE_CURVE('',#3023,#3014,#198,.T.);
#3782=EDGE_CURVE('',#3024,#2982,#1890,.T.);
#3783=EDGE_CURVE('',#3024,#3025,#199,.T.);
#3784=EDGE_CURVE('',#3025,#3018,#200,.T.);
#3785=EDGE_CURVE('',#2981,#3026,#1891,.T.);
#3786=EDGE_CURVE('',#3027,#3026,#201,.T.);
#3787=EDGE_CURVE('',#3027,#3028,#202,.T.);
#3788=EDGE_CURVE('',#3029,#3028,#203,.T.);
#3789=EDGE_CURVE('',#3029,#3030,#1892,.T.);
#3790=EDGE_CURVE('',#3031,#3030,#204,.T.);
#3791=EDGE_CURVE('',#3031,#3032,#205,.T.);
#3792=EDGE_CURVE('',#3033,#3032,#206,.T.);
#3793=EDGE_CURVE('',#3033,#2964,#1893,.T.);
#3794=EDGE_CURVE('',#3021,#3034,#207,.T.);
#3795=EDGE_CURVE('',#3034,#3035,#208,.T.);
#3796=EDGE_CURVE('',#2967,#3035,#1894,.T.);
#3797=EDGE_CURVE('',#3017,#3036,#209,.T.);
#3798=EDGE_CURVE('',#2971,#3036,#1895,.T.);
#3799=EDGE_CURVE('',#3013,#3037,#210,.T.);
#3800=EDGE_CURVE('',#2975,#3037,#1896,.T.);
#3801=EDGE_CURVE('',#3038,#3039,#211,.T.);
#3802=EDGE_CURVE('',#3039,#3040,#212,.T.);
#3803=EDGE_CURVE('',#3040,#3041,#1897,.T.);
#3804=EDGE_CURVE('',#3041,#3042,#213,.T.);
#3805=EDGE_CURVE('',#3042,#3043,#214,.T.);
#3806=EDGE_CURVE('',#3038,#3043,#1898,.T.);
#3807=EDGE_CURVE('',#3044,#3044,#2701,.T.);
#3808=EDGE_CURVE('',#3044,#2991,#1899,.T.);
#3809=EDGE_CURVE('',#2947,#2990,#1900,.T.);
#3810=EDGE_CURVE('',#3038,#3045,#215,.T.);
#3811=EDGE_CURVE('',#3046,#3043,#216,.T.);
#3812=EDGE_CURVE('',#3047,#3046,#217,.T.);
#3813=EDGE_CURVE('',#3048,#3047,#1901,.T.);
#3814=EDGE_CURVE('',#3045,#3048,#218,.T.);
#3815=EDGE_CURVE('',#3006,#2998,#219,.T.);
#3816=EDGE_CURVE('',#3045,#3049,#220,.T.);
#3817=EDGE_CURVE('',#3049,#3039,#221,.T.);
#3818=EDGE_CURVE('',#2999,#3005,#222,.T.);
#3819=EDGE_CURVE('',#3050,#3048,#223,.T.);
#3820=EDGE_CURVE('',#3049,#3050,#2702,.F.);
#3821=EDGE_CURVE('',#3004,#3000,#224,.T.);
#3822=EDGE_CURVE('',#3047,#3051,#225,.T.);
#3823=EDGE_CURVE('',#3051,#3050,#1902,.T.);
#3824=EDGE_CURVE('',#3001,#3003,#226,.T.);
#3825=EDGE_CURVE('',#3042,#3052,#227,.T.);
#3826=EDGE_CURVE('',#3052,#3046,#228,.T.);
#3827=EDGE_CURVE('',#3053,#3037,#229,.T.);
#3828=EDGE_CURVE('',#3054,#3053,#230,.T.);
#3829=EDGE_CURVE('',#3055,#3054,#1903,.T.);
#3830=EDGE_CURVE('',#3056,#3055,#231,.T.);
#3831=EDGE_CURVE('',#3022,#3056,#232,.T.);
#3832=EDGE_CURVE('',#3012,#3053,#233,.T.);
#3833=EDGE_CURVE('',#3054,#3011,#234,.T.);
#3834=EDGE_CURVE('',#3010,#3055,#235,.T.);
#3835=EDGE_CURVE('',#3056,#3009,#236,.T.);
#3836=EDGE_CURVE('',#3057,#3036,#237,.T.);
#3837=EDGE_CURVE('',#2939,#3057,#238,.T.);
#3838=EDGE_CURVE('',#3058,#2938,#239,.T.);
#3839=EDGE_CURVE('',#3023,#3058,#240,.T.);
#3840=EDGE_CURVE('',#3016,#3057,#241,.T.);
#3841=EDGE_CURVE('',#3058,#3015,#242,.T.);
#3842=EDGE_CURVE('',#3059,#3035,#243,.T.);
#3843=EDGE_CURVE('',#3060,#3059,#244,.T.);
#3844=EDGE_CURVE('',#3061,#3060,#1904,.T.);
#3845=EDGE_CURVE('',#3062,#3061,#245,.T.);
#3846=EDGE_CURVE('',#3024,#3062,#246,.T.);
#3847=EDGE_CURVE('',#3034,#3063,#247,.T.);
#3848=EDGE_CURVE('',#3063,#3059,#248,.T.);
#3849=EDGE_CURVE('',#3064,#3063,#2703,.F.);
#3850=EDGE_CURVE('',#3060,#3064,#249,.T.);
#3851=EDGE_CURVE('',#3064,#3065,#1905,.T.);
#3852=EDGE_CURVE('',#3065,#3061,#250,.T.);
#3853=EDGE_CURVE('',#3062,#3066,#251,.T.);
#3854=EDGE_CURVE('',#3066,#3025,#252,.T.);
#3855=EDGE_CURVE('',#3066,#3065,#2704,.F.);
#3856=EDGE_CURVE('',#3065,#3019,#2705,.F.);
#3857=EDGE_CURVE('',#3019,#3066,#2706,.F.);
#3858=EDGE_CURVE('',#3051,#3052,#2707,.F.);
#3859=EDGE_CURVE('',#3052,#3067,#2708,.F.);
#3860=EDGE_CURVE('',#3067,#3051,#2709,.F.);
#3861=EDGE_CURVE('',#3063,#3020,#2710,.F.);
#3862=EDGE_CURVE('',#3020,#3064,#2711,.F.);
#3863=EDGE_CURVE('',#3068,#3049,#2712,.F.);
#3864=EDGE_CURVE('',#3050,#3068,#2713,.F.);
#3865=EDGE_CURVE('',#3068,#3067,#1906,.T.);
#3866=EDGE_CURVE('',#3040,#3068,#253,.T.);
#3867=EDGE_CURVE('',#3067,#3041,#254,.T.);
#3868=EDGE_CURVE('',#3069,#3070,#2714,.F.);
#3869=EDGE_CURVE('',#3071,#3069,#2715,.F.);
#3870=EDGE_CURVE('',#3070,#3071,#2716,.F.);
#3871=EDGE_CURVE('',#3072,#3073,#2717,.F.);
#3872=EDGE_CURVE('',#3074,#3072,#2718,.F.);
#3873=EDGE_CURVE('',#3073,#3074,#2719,.F.);
#3874=EDGE_CURVE('',#3075,#3076,#2720,.F.);
#3875=EDGE_CURVE('',#3077,#3075,#2721,.F.);
#3876=EDGE_CURVE('',#3076,#3077,#2722,.F.);
#3877=EDGE_CURVE('',#3070,#3077,#1907,.T.);
#3878=EDGE_CURVE('',#3075,#3069,#1908,.T.);
#3879=EDGE_CURVE('',#3032,#3076,#255,.T.);
#3880=EDGE_CURVE('',#3077,#3033,#256,.T.);
#3881=EDGE_CURVE('',#3078,#3079,#2723,.F.);
#3882=EDGE_CURVE('',#3080,#3078,#2724,.F.);
#3883=EDGE_CURVE('',#3079,#3080,#2725,.F.);
#3884=EDGE_CURVE('',#3078,#3074,#1909,.T.);
#3885=EDGE_CURVE('',#3072,#3080,#1910,.T.);
#3886=EDGE_CURVE('',#3076,#3079,#257,.T.);
#3887=EDGE_CURVE('',#3080,#3075,#258,.T.);
#3888=EDGE_CURVE('',#3030,#3078,#259,.T.);
#3889=EDGE_CURVE('',#3079,#3031,#260,.T.);
#3890=EDGE_CURVE('',#3028,#3073,#261,.T.);
#3891=EDGE_CURVE('',#3074,#3029,#262,.T.);
#3892=EDGE_CURVE('',#3073,#3071,#263,.T.);
#3893=EDGE_CURVE('',#3069,#3072,#264,.T.);
#3894=EDGE_CURVE('',#3026,#3070,#265,.T.);
#3895=EDGE_CURVE('',#3071,#3027,#266,.T.);
#4890=ORIENTED_EDGE('',*,*,#3670,.T.);
#4891=ORIENTED_EDGE('',*,*,#3671,.T.);
#4892=ORIENTED_EDGE('',*,*,#3672,.T.);
#4893=ORIENTED_EDGE('',*,*,#3673,.F.);
#4894=ORIENTED_EDGE('',*,*,#3674,.T.);
#4895=ORIENTED_EDGE('',*,*,#3675,.T.);
#4896=ORIENTED_EDGE('',*,*,#3676,.T.);
#4897=ORIENTED_EDGE('',*,*,#3677,.F.);
#4898=ORIENTED_EDGE('',*,*,#3678,.T.);
#4899=ORIENTED_EDGE('',*,*,#3679,.T.);
#4900=ORIENTED_EDGE('',*,*,#3680,.T.);
#4901=ORIENTED_EDGE('',*,*,#3681,.F.);
#4902=ORIENTED_EDGE('',*,*,#3682,.T.);
#4903=ORIENTED_EDGE('',*,*,#3683,.F.);
#4904=ORIENTED_EDGE('',*,*,#3682,.F.);
#4905=ORIENTED_EDGE('',*,*,#3684,.F.);
#4906=ORIENTED_EDGE('',*,*,#3685,.T.);
#4907=ORIENTED_EDGE('',*,*,#3679,.F.);
#4908=ORIENTED_EDGE('',*,*,#3685,.F.);
#4909=ORIENTED_EDGE('',*,*,#3686,.F.);
#4910=ORIENTED_EDGE('',*,*,#3687,.T.);
#4911=ORIENTED_EDGE('',*,*,#3678,.F.);
#4912=ORIENTED_EDGE('',*,*,#3687,.F.);
#4913=ORIENTED_EDGE('',*,*,#3688,.F.);
#4914=ORIENTED_EDGE('',*,*,#3689,.T.);
#4915=ORIENTED_EDGE('',*,*,#3690,.F.);
#4916=ORIENTED_EDGE('',*,*,#3689,.F.);
#4917=ORIENTED_EDGE('',*,*,#3691,.F.);
#4918=ORIENTED_EDGE('',*,*,#3692,.T.);
#4919=ORIENTED_EDGE('',*,*,#3693,.T.);
#4920=ORIENTED_EDGE('',*,*,#3692,.F.);
#4921=ORIENTED_EDGE('',*,*,#3693,.F.);
#4922=ORIENTED_EDGE('',*,*,#3694,.F.);
#4923=ORIENTED_EDGE('',*,*,#3695,.F.);
#4924=ORIENTED_EDGE('',*,*,#3696,.T.);
#4925=ORIENTED_EDGE('',*,*,#3697,.T.);
#4926=ORIENTED_EDGE('',*,*,#3696,.F.);
#4927=ORIENTED_EDGE('',*,*,#3697,.F.);
#4928=ORIENTED_EDGE('',*,*,#3698,.F.);
#4929=ORIENTED_EDGE('',*,*,#3694,.T.);
#4930=ORIENTED_EDGE('',*,*,#3699,.T.);
#4931=ORIENTED_EDGE('',*,*,#3700,.F.);
#4932=ORIENTED_EDGE('',*,*,#3699,.F.);
#4933=ORIENTED_EDGE('',*,*,#3698,.T.);
#4934=ORIENTED_EDGE('',*,*,#3701,.T.);
#4935=ORIENTED_EDGE('',*,*,#3702,.F.);
#4936=ORIENTED_EDGE('',*,*,#3701,.F.);
#4937=ORIENTED_EDGE('',*,*,#3703,.F.);
#4938=ORIENTED_EDGE('',*,*,#3704,.F.);
#4939=ORIENTED_EDGE('',*,*,#3705,.F.);
#4940=ORIENTED_EDGE('',*,*,#3706,.T.);
#4941=ORIENTED_EDGE('',*,*,#3707,.F.);
#4942=ORIENTED_EDGE('',*,*,#3708,.T.);
#4943=ORIENTED_EDGE('',*,*,#3709,.F.);
#4944=ORIENTED_EDGE('',*,*,#3710,.F.);
#4945=ORIENTED_EDGE('',*,*,#3711,.F.);
#4946=ORIENTED_EDGE('',*,*,#3712,.T.);
#4947=ORIENTED_EDGE('',*,*,#3713,.F.);
#4948=ORIENTED_EDGE('',*,*,#3714,.F.);
#4949=ORIENTED_EDGE('',*,*,#3715,.F.);
#4950=ORIENTED_EDGE('',*,*,#3716,.T.);
#4951=ORIENTED_EDGE('',*,*,#3717,.F.);
#4952=ORIENTED_EDGE('',*,*,#3718,.F.);
#4953=ORIENTED_EDGE('',*,*,#3719,.F.);
#4954=ORIENTED_EDGE('',*,*,#3720,.T.);
#4955=ORIENTED_EDGE('',*,*,#3721,.F.);
#4956=ORIENTED_EDGE('',*,*,#3722,.F.);
#4957=ORIENTED_EDGE('',*,*,#3723,.F.);
#4958=ORIENTED_EDGE('',*,*,#3724,.F.);
#4959=ORIENTED_EDGE('',*,*,#3725,.F.);
#4960=ORIENTED_EDGE('',*,*,#3726,.T.);
#4961=ORIENTED_EDGE('',*,*,#3727,.F.);
#4962=ORIENTED_EDGE('',*,*,#3728,.F.);
#4963=ORIENTED_EDGE('',*,*,#3729,.F.);
#4964=ORIENTED_EDGE('',*,*,#3730,.T.);
#4965=ORIENTED_EDGE('',*,*,#3731,.F.);
#4966=ORIENTED_EDGE('',*,*,#3700,.T.);
#4967=ORIENTED_EDGE('',*,*,#3732,.F.);
#4968=ORIENTED_EDGE('',*,*,#3702,.T.);
#4969=ORIENTED_EDGE('',*,*,#3733,.F.);
#4970=ORIENTED_EDGE('',*,*,#3706,.F.);
#4971=ORIENTED_EDGE('',*,*,#3734,.F.);
#4972=ORIENTED_EDGE('',*,*,#3720,.F.);
#4973=ORIENTED_EDGE('',*,*,#3735,.F.);
#4974=ORIENTED_EDGE('',*,*,#3726,.F.);
#4975=ORIENTED_EDGE('',*,*,#3736,.F.);
#4976=ORIENTED_EDGE('',*,*,#3708,.F.);
#4977=ORIENTED_EDGE('',*,*,#3737,.F.);
#4978=ORIENTED_EDGE('',*,*,#3730,.F.);
#4979=ORIENTED_EDGE('',*,*,#3738,.F.);
#4980=ORIENTED_EDGE('',*,*,#3712,.F.);
#4981=ORIENTED_EDGE('',*,*,#3739,.F.);
#4982=ORIENTED_EDGE('',*,*,#3740,.F.);
#4983=ORIENTED_EDGE('',*,*,#3741,.F.);
#4984=ORIENTED_EDGE('',*,*,#3716,.F.);
#4985=ORIENTED_EDGE('',*,*,#3742,.F.);
#4986=ORIENTED_EDGE('',*,*,#3743,.F.);
#4987=ORIENTED_EDGE('',*,*,#3744,.F.);
#4988=ORIENTED_EDGE('',*,*,#3740,.T.);
#4989=ORIENTED_EDGE('',*,*,#3745,.T.);
#4990=ORIENTED_EDGE('',*,*,#3746,.F.);
#4991=ORIENTED_EDGE('',*,*,#3747,.F.);
#4992=ORIENTED_EDGE('',*,*,#3748,.F.);
#4993=ORIENTED_EDGE('',*,*,#3749,.F.);
#4994=ORIENTED_EDGE('',*,*,#3750,.F.);
#4995=ORIENTED_EDGE('',*,*,#3717,.T.);
#4996=ORIENTED_EDGE('',*,*,#3741,.T.);
#4997=ORIENTED_EDGE('',*,*,#3744,.T.);
#4998=ORIENTED_EDGE('',*,*,#3751,.T.);
#4999=ORIENTED_EDGE('',*,*,#3752,.F.);
#5000=ORIENTED_EDGE('',*,*,#3753,.F.);
#5001=ORIENTED_EDGE('',*,*,#3754,.F.);
#5002=ORIENTED_EDGE('',*,*,#3755,.F.);
#5003=ORIENTED_EDGE('',*,*,#3756,.F.);
#5004=ORIENTED_EDGE('',*,*,#3757,.T.);
#5005=ORIENTED_EDGE('',*,*,#3713,.T.);
#5006=ORIENTED_EDGE('',*,*,#3738,.T.);
#5007=ORIENTED_EDGE('',*,*,#3729,.T.);
#5008=ORIENTED_EDGE('',*,*,#3758,.T.);
#5009=ORIENTED_EDGE('',*,*,#3759,.F.);
#5010=ORIENTED_EDGE('',*,*,#3760,.F.);
#5011=ORIENTED_EDGE('',*,*,#3761,.F.);
#5012=ORIENTED_EDGE('',*,*,#3762,.F.);
#5013=ORIENTED_EDGE('',*,*,#3763,.F.);
#5014=ORIENTED_EDGE('',*,*,#3764,.T.);
#5015=ORIENTED_EDGE('',*,*,#3709,.T.);
#5016=ORIENTED_EDGE('',*,*,#3736,.T.);
#5017=ORIENTED_EDGE('',*,*,#3725,.T.);
#5018=ORIENTED_EDGE('',*,*,#3765,.T.);
#5019=ORIENTED_EDGE('',*,*,#3766,.F.);
#5020=ORIENTED_EDGE('',*,*,#3767,.F.);
#5021=ORIENTED_EDGE('',*,*,#3675,.F.);
#5022=ORIENTED_EDGE('',*,*,#3768,.F.);
#5023=ORIENTED_EDGE('',*,*,#3769,.F.);
#5024=ORIENTED_EDGE('',*,*,#3770,.T.);
#5025=ORIENTED_EDGE('',*,*,#3703,.T.);
#5026=ORIENTED_EDGE('',*,*,#3733,.T.);
#5027=ORIENTED_EDGE('',*,*,#3719,.T.);
#5028=ORIENTED_EDGE('',*,*,#3771,.F.);
#5029=ORIENTED_EDGE('',*,*,#3772,.T.);
#5030=ORIENTED_EDGE('',*,*,#3773,.T.);
#5031=ORIENTED_EDGE('',*,*,#3774,.T.);
#5032=ORIENTED_EDGE('',*,*,#3775,.F.);
#5033=ORIENTED_EDGE('',*,*,#3718,.T.);
#5034=ORIENTED_EDGE('',*,*,#3757,.F.);
#5035=ORIENTED_EDGE('',*,*,#3776,.T.);
#5036=ORIENTED_EDGE('',*,*,#3745,.F.);
#5037=ORIENTED_EDGE('',*,*,#3777,.T.);
#5038=ORIENTED_EDGE('',*,*,#3751,.F.);
#5039=ORIENTED_EDGE('',*,*,#3743,.T.);
#5040=ORIENTED_EDGE('',*,*,#3778,.F.);
#5041=ORIENTED_EDGE('',*,*,#3779,.T.);
#5042=ORIENTED_EDGE('',*,*,#3758,.F.);
#5043=ORIENTED_EDGE('',*,*,#3728,.T.);
#5044=ORIENTED_EDGE('',*,*,#3780,.F.);
#5045=ORIENTED_EDGE('',*,*,#3781,.T.);
#5046=ORIENTED_EDGE('',*,*,#3765,.F.);
#5047=ORIENTED_EDGE('',*,*,#3724,.T.);
#5048=ORIENTED_EDGE('',*,*,#3782,.F.);
#5049=ORIENTED_EDGE('',*,*,#3783,.T.);
#5050=ORIENTED_EDGE('',*,*,#3784,.T.);
#5051=ORIENTED_EDGE('',*,*,#3771,.T.);
#5052=ORIENTED_EDGE('',*,*,#3722,.T.);
#5053=ORIENTED_EDGE('',*,*,#3785,.T.);
#5054=ORIENTED_EDGE('',*,*,#3786,.F.);
#5055=ORIENTED_EDGE('',*,*,#3787,.T.);
#5056=ORIENTED_EDGE('',*,*,#3788,.F.);
#5057=ORIENTED_EDGE('',*,*,#3789,.T.);
#5058=ORIENTED_EDGE('',*,*,#3790,.F.);
#5059=ORIENTED_EDGE('',*,*,#3791,.T.);
#5060=ORIENTED_EDGE('',*,*,#3792,.F.);
#5061=ORIENTED_EDGE('',*,*,#3793,.T.);
#5062=ORIENTED_EDGE('',*,*,#3704,.T.);
#5063=ORIENTED_EDGE('',*,*,#3775,.T.);
#5064=ORIENTED_EDGE('',*,*,#3794,.T.);
#5065=ORIENTED_EDGE('',*,*,#3795,.T.);
#5066=ORIENTED_EDGE('',*,*,#3796,.F.);
#5067=ORIENTED_EDGE('',*,*,#3710,.T.);
#5068=ORIENTED_EDGE('',*,*,#3770,.F.);
#5069=ORIENTED_EDGE('',*,*,#3797,.T.);
#5070=ORIENTED_EDGE('',*,*,#3798,.F.);
#5071=ORIENTED_EDGE('',*,*,#3714,.T.);
#5072=ORIENTED_EDGE('',*,*,#3764,.F.);
#5073=ORIENTED_EDGE('',*,*,#3799,.T.);
#5074=ORIENTED_EDGE('',*,*,#3800,.F.);
#5075=ORIENTED_EDGE('',*,*,#3801,.T.);
#5076=ORIENTED_EDGE('',*,*,#3802,.T.);
#5077=ORIENTED_EDGE('',*,*,#3803,.T.);
#5078=ORIENTED_EDGE('',*,*,#3804,.T.);
#5079=ORIENTED_EDGE('',*,*,#3805,.T.);
#5080=ORIENTED_EDGE('',*,*,#3806,.F.);
#5081=ORIENTED_EDGE('',*,*,#3807,.F.);
#5082=ORIENTED_EDGE('',*,*,#3808,.T.);
#5083=ORIENTED_EDGE('',*,*,#3732,.T.);
#5084=ORIENTED_EDGE('',*,*,#3808,.F.);
#5085=ORIENTED_EDGE('',*,*,#3680,.F.);
#5086=ORIENTED_EDGE('',*,*,#3809,.T.);
#5087=ORIENTED_EDGE('',*,*,#3731,.T.);
#5088=ORIENTED_EDGE('',*,*,#3809,.F.);
#5089=ORIENTED_EDGE('',*,*,#3810,.F.);
#5090=ORIENTED_EDGE('',*,*,#3806,.T.);
#5091=ORIENTED_EDGE('',*,*,#3811,.F.);
#5092=ORIENTED_EDGE('',*,*,#3812,.F.);
#5093=ORIENTED_EDGE('',*,*,#3813,.F.);
#5094=ORIENTED_EDGE('',*,*,#3814,.F.);
#5095=ORIENTED_EDGE('',*,*,#3746,.T.);
#5096=ORIENTED_EDGE('',*,*,#3776,.F.);
#5097=ORIENTED_EDGE('',*,*,#3756,.T.);
#5098=ORIENTED_EDGE('',*,*,#3815,.T.);
#5099=ORIENTED_EDGE('',*,*,#3810,.T.);
#5100=ORIENTED_EDGE('',*,*,#3816,.T.);
#5101=ORIENTED_EDGE('',*,*,#3817,.T.);
#5102=ORIENTED_EDGE('',*,*,#3801,.F.);
#5103=ORIENTED_EDGE('',*,*,#3747,.T.);
#5104=ORIENTED_EDGE('',*,*,#3815,.F.);
#5105=ORIENTED_EDGE('',*,*,#3755,.T.);
#5106=ORIENTED_EDGE('',*,*,#3818,.F.);
#5107=ORIENTED_EDGE('',*,*,#3814,.T.);
#5108=ORIENTED_EDGE('',*,*,#3819,.F.);
#5109=ORIENTED_EDGE('',*,*,#3820,.F.);
#5110=ORIENTED_EDGE('',*,*,#3816,.F.);
#5111=ORIENTED_EDGE('',*,*,#3748,.T.);
#5112=ORIENTED_EDGE('',*,*,#3818,.T.);
#5113=ORIENTED_EDGE('',*,*,#3754,.T.);
#5114=ORIENTED_EDGE('',*,*,#3821,.T.);
#5115=ORIENTED_EDGE('',*,*,#3683,.T.);
#5116=ORIENTED_EDGE('',*,*,#3690,.T.);
#5117=ORIENTED_EDGE('',*,*,#3807,.T.);
#5118=ORIENTED_EDGE('',*,*,#3813,.T.);
#5119=ORIENTED_EDGE('',*,*,#3822,.T.);
#5120=ORIENTED_EDGE('',*,*,#3823,.T.);
#5121=ORIENTED_EDGE('',*,*,#3819,.T.);
#5122=ORIENTED_EDGE('',*,*,#3749,.T.);
#5123=ORIENTED_EDGE('',*,*,#3821,.F.);
#5124=ORIENTED_EDGE('',*,*,#3753,.T.);
#5125=ORIENTED_EDGE('',*,*,#3824,.F.);
#5126=ORIENTED_EDGE('',*,*,#3750,.T.);
#5127=ORIENTED_EDGE('',*,*,#3824,.T.);
#5128=ORIENTED_EDGE('',*,*,#3752,.T.);
#5129=ORIENTED_EDGE('',*,*,#3777,.F.);
#5130=ORIENTED_EDGE('',*,*,#3811,.T.);
#5131=ORIENTED_EDGE('',*,*,#3805,.F.);
#5132=ORIENTED_EDGE('',*,*,#3825,.T.);
#5133=ORIENTED_EDGE('',*,*,#3826,.T.);
#5134=ORIENTED_EDGE('',*,*,#3715,.T.);
#5135=ORIENTED_EDGE('',*,*,#3800,.T.);
#5136=ORIENTED_EDGE('',*,*,#3827,.F.);
#5137=ORIENTED_EDGE('',*,*,#3828,.F.);
#5138=ORIENTED_EDGE('',*,*,#3829,.F.);
#5139=ORIENTED_EDGE('',*,*,#3830,.F.);
#5140=ORIENTED_EDGE('',*,*,#3831,.F.);
#5141=ORIENTED_EDGE('',*,*,#3778,.T.);
#5142=ORIENTED_EDGE('',*,*,#3742,.T.);
#5143=ORIENTED_EDGE('',*,*,#3739,.T.);
#5144=ORIENTED_EDGE('',*,*,#3827,.T.);
#5145=ORIENTED_EDGE('',*,*,#3799,.F.);
#5146=ORIENTED_EDGE('',*,*,#3763,.T.);
#5147=ORIENTED_EDGE('',*,*,#3832,.T.);
#5148=ORIENTED_EDGE('',*,*,#3828,.T.);
#5149=ORIENTED_EDGE('',*,*,#3832,.F.);
#5150=ORIENTED_EDGE('',*,*,#3762,.T.);
#5151=ORIENTED_EDGE('',*,*,#3833,.F.);
#5152=ORIENTED_EDGE('',*,*,#3829,.T.);
#5153=ORIENTED_EDGE('',*,*,#3833,.T.);
#5154=ORIENTED_EDGE('',*,*,#3761,.T.);
#5155=ORIENTED_EDGE('',*,*,#3834,.T.);
#5156=ORIENTED_EDGE('',*,*,#3830,.T.);
#5157=ORIENTED_EDGE('',*,*,#3834,.F.);
#5158=ORIENTED_EDGE('',*,*,#3760,.T.);
#5159=ORIENTED_EDGE('',*,*,#3835,.F.);
#5160=ORIENTED_EDGE('',*,*,#3831,.T.);
#5161=ORIENTED_EDGE('',*,*,#3835,.T.);
#5162=ORIENTED_EDGE('',*,*,#3759,.T.);
#5163=ORIENTED_EDGE('',*,*,#3779,.F.);
#5164=ORIENTED_EDGE('',*,*,#3711,.T.);
#5165=ORIENTED_EDGE('',*,*,#3798,.T.);
#5166=ORIENTED_EDGE('',*,*,#3836,.F.);
#5167=ORIENTED_EDGE('',*,*,#3837,.F.);
#5168=ORIENTED_EDGE('',*,*,#3671,.F.);
#5169=ORIENTED_EDGE('',*,*,#3838,.F.);
#5170=ORIENTED_EDGE('',*,*,#3839,.F.);
#5171=ORIENTED_EDGE('',*,*,#3780,.T.);
#5172=ORIENTED_EDGE('',*,*,#3727,.T.);
#5173=ORIENTED_EDGE('',*,*,#3737,.T.);
#5174=ORIENTED_EDGE('',*,*,#3836,.T.);
#5175=ORIENTED_EDGE('',*,*,#3797,.F.);
#5176=ORIENTED_EDGE('',*,*,#3769,.T.);
#5177=ORIENTED_EDGE('',*,*,#3840,.T.);
#5178=ORIENTED_EDGE('',*,*,#3673,.T.);
#5179=ORIENTED_EDGE('',*,*,#3672,.F.);
#5180=ORIENTED_EDGE('',*,*,#3837,.T.);
#5181=ORIENTED_EDGE('',*,*,#3840,.F.);
#5182=ORIENTED_EDGE('',*,*,#3768,.T.);
#5183=ORIENTED_EDGE('',*,*,#3674,.F.);
#5184=ORIENTED_EDGE('',*,*,#3677,.T.);
#5185=ORIENTED_EDGE('',*,*,#3676,.F.);
#5186=ORIENTED_EDGE('',*,*,#3767,.T.);
#5187=ORIENTED_EDGE('',*,*,#3841,.F.);
#5188=ORIENTED_EDGE('',*,*,#3838,.T.);
#5189=ORIENTED_EDGE('',*,*,#3670,.F.);
#5190=ORIENTED_EDGE('',*,*,#3839,.T.);
#5191=ORIENTED_EDGE('',*,*,#3841,.T.);
#5192=ORIENTED_EDGE('',*,*,#3766,.T.);
#5193=ORIENTED_EDGE('',*,*,#3781,.F.);
#5194=ORIENTED_EDGE('',*,*,#3707,.T.);
#5195=ORIENTED_EDGE('',*,*,#3796,.T.);
#5196=ORIENTED_EDGE('',*,*,#3842,.F.);
#5197=ORIENTED_EDGE('',*,*,#3843,.F.);
#5198=ORIENTED_EDGE('',*,*,#3844,.F.);
#5199=ORIENTED_EDGE('',*,*,#3845,.F.);
#5200=ORIENTED_EDGE('',*,*,#3846,.F.);
#5201=ORIENTED_EDGE('',*,*,#3782,.T.);
#5202=ORIENTED_EDGE('',*,*,#3723,.T.);
#5203=ORIENTED_EDGE('',*,*,#3735,.T.);
#5204=ORIENTED_EDGE('',*,*,#3842,.T.);
#5205=ORIENTED_EDGE('',*,*,#3795,.F.);
#5206=ORIENTED_EDGE('',*,*,#3847,.T.);
#5207=ORIENTED_EDGE('',*,*,#3848,.T.);
#5208=ORIENTED_EDGE('',*,*,#3843,.T.);
#5209=ORIENTED_EDGE('',*,*,#3848,.F.);
#5210=ORIENTED_EDGE('',*,*,#3849,.F.);
#5211=ORIENTED_EDGE('',*,*,#3850,.F.);
#5212=ORIENTED_EDGE('',*,*,#3844,.T.);
#5213=ORIENTED_EDGE('',*,*,#3850,.T.);
#5214=ORIENTED_EDGE('',*,*,#3851,.T.);
#5215=ORIENTED_EDGE('',*,*,#3852,.T.);
#5216=ORIENTED_EDGE('',*,*,#3846,.T.);
#5217=ORIENTED_EDGE('',*,*,#3853,.T.);
#5218=ORIENTED_EDGE('',*,*,#3854,.T.);
#5219=ORIENTED_EDGE('',*,*,#3783,.F.);
#5220=ORIENTED_EDGE('',*,*,#3845,.T.);
#5221=ORIENTED_EDGE('',*,*,#3852,.F.);
#5222=ORIENTED_EDGE('',*,*,#3855,.F.);
#5223=ORIENTED_EDGE('',*,*,#3853,.F.);
#5224=ORIENTED_EDGE('',*,*,#3856,.T.);
#5225=ORIENTED_EDGE('',*,*,#3857,.T.);
#5226=ORIENTED_EDGE('',*,*,#3855,.T.);
#5227=ORIENTED_EDGE('',*,*,#3858,.T.);
#5228=ORIENTED_EDGE('',*,*,#3859,.T.);
#5229=ORIENTED_EDGE('',*,*,#3860,.T.);
#5230=ORIENTED_EDGE('',*,*,#3849,.T.);
#5231=ORIENTED_EDGE('',*,*,#3861,.T.);
#5232=ORIENTED_EDGE('',*,*,#3862,.T.);
#5233=ORIENTED_EDGE('',*,*,#3856,.F.);
#5234=ORIENTED_EDGE('',*,*,#3851,.F.);
#5235=ORIENTED_EDGE('',*,*,#3862,.F.);
#5236=ORIENTED_EDGE('',*,*,#3773,.F.);
#5237=ORIENTED_EDGE('',*,*,#3794,.F.);
#5238=ORIENTED_EDGE('',*,*,#3774,.F.);
#5239=ORIENTED_EDGE('',*,*,#3861,.F.);
#5240=ORIENTED_EDGE('',*,*,#3847,.F.);
#5241=ORIENTED_EDGE('',*,*,#3863,.T.);
#5242=ORIENTED_EDGE('',*,*,#3820,.T.);
#5243=ORIENTED_EDGE('',*,*,#3864,.T.);
#5244=ORIENTED_EDGE('',*,*,#3864,.F.);
#5245=ORIENTED_EDGE('',*,*,#3823,.F.);
#5246=ORIENTED_EDGE('',*,*,#3860,.F.);
#5247=ORIENTED_EDGE('',*,*,#3865,.F.);
#5248=ORIENTED_EDGE('',*,*,#3802,.F.);
#5249=ORIENTED_EDGE('',*,*,#3817,.F.);
#5250=ORIENTED_EDGE('',*,*,#3863,.F.);
#5251=ORIENTED_EDGE('',*,*,#3866,.F.);
#5252=ORIENTED_EDGE('',*,*,#3804,.F.);
#5253=ORIENTED_EDGE('',*,*,#3867,.F.);
#5254=ORIENTED_EDGE('',*,*,#3859,.F.);
#5255=ORIENTED_EDGE('',*,*,#3825,.F.);
#5256=ORIENTED_EDGE('',*,*,#3812,.T.);
#5257=ORIENTED_EDGE('',*,*,#3826,.F.);
#5258=ORIENTED_EDGE('',*,*,#3858,.F.);
#5259=ORIENTED_EDGE('',*,*,#3822,.F.);
#5260=ORIENTED_EDGE('',*,*,#3784,.F.);
#5261=ORIENTED_EDGE('',*,*,#3854,.F.);
#5262=ORIENTED_EDGE('',*,*,#3857,.F.);
#5263=ORIENTED_EDGE('',*,*,#3772,.F.);
#5264=ORIENTED_EDGE('',*,*,#3866,.T.);
#5265=ORIENTED_EDGE('',*,*,#3865,.T.);
#5266=ORIENTED_EDGE('',*,*,#3867,.T.);
#5267=ORIENTED_EDGE('',*,*,#3803,.F.);
#5268=ORIENTED_EDGE('',*,*,#3868,.F.);
#5269=ORIENTED_EDGE('',*,*,#3869,.F.);
#5270=ORIENTED_EDGE('',*,*,#3870,.F.);
#5271=ORIENTED_EDGE('',*,*,#3871,.F.);
#5272=ORIENTED_EDGE('',*,*,#3872,.F.);
#5273=ORIENTED_EDGE('',*,*,#3873,.F.);
#5274=ORIENTED_EDGE('',*,*,#3874,.F.);
#5275=ORIENTED_EDGE('',*,*,#3875,.F.);
#5276=ORIENTED_EDGE('',*,*,#3876,.F.);
#5277=ORIENTED_EDGE('',*,*,#3868,.T.);
#5278=ORIENTED_EDGE('',*,*,#3877,.T.);
#5279=ORIENTED_EDGE('',*,*,#3875,.T.);
#5280=ORIENTED_EDGE('',*,*,#3878,.T.);
#5281=ORIENTED_EDGE('',*,*,#3792,.T.);
#5282=ORIENTED_EDGE('',*,*,#3879,.T.);
#5283=ORIENTED_EDGE('',*,*,#3876,.T.);
#5284=ORIENTED_EDGE('',*,*,#3880,.T.);
#5285=ORIENTED_EDGE('',*,*,#3881,.F.);
#5286=ORIENTED_EDGE('',*,*,#3882,.F.);
#5287=ORIENTED_EDGE('',*,*,#3883,.F.);
#5288=ORIENTED_EDGE('',*,*,#3882,.T.);
#5289=ORIENTED_EDGE('',*,*,#3884,.T.);
#5290=ORIENTED_EDGE('',*,*,#3872,.T.);
#5291=ORIENTED_EDGE('',*,*,#3885,.T.);
#5292=ORIENTED_EDGE('',*,*,#3874,.T.);
#5293=ORIENTED_EDGE('',*,*,#3886,.T.);
#5294=ORIENTED_EDGE('',*,*,#3883,.T.);
#5295=ORIENTED_EDGE('',*,*,#3887,.T.);
#5296=ORIENTED_EDGE('',*,*,#3790,.T.);
#5297=ORIENTED_EDGE('',*,*,#3888,.T.);
#5298=ORIENTED_EDGE('',*,*,#3881,.T.);
#5299=ORIENTED_EDGE('',*,*,#3889,.T.);
#5300=ORIENTED_EDGE('',*,*,#3788,.T.);
#5301=ORIENTED_EDGE('',*,*,#3890,.T.);
#5302=ORIENTED_EDGE('',*,*,#3873,.T.);
#5303=ORIENTED_EDGE('',*,*,#3891,.T.);
#5304=ORIENTED_EDGE('',*,*,#3871,.T.);
#5305=ORIENTED_EDGE('',*,*,#3892,.T.);
#5306=ORIENTED_EDGE('',*,*,#3869,.T.);
#5307=ORIENTED_EDGE('',*,*,#3893,.T.);
#5308=ORIENTED_EDGE('',*,*,#3786,.T.);
#5309=ORIENTED_EDGE('',*,*,#3894,.T.);
#5310=ORIENTED_EDGE('',*,*,#3870,.T.);
#5311=ORIENTED_EDGE('',*,*,#3895,.T.);
#5312=ORIENTED_EDGE('',*,*,#3889,.F.);
#5313=ORIENTED_EDGE('',*,*,#3886,.F.);
#5314=ORIENTED_EDGE('',*,*,#3879,.F.);
#5315=ORIENTED_EDGE('',*,*,#3791,.F.);
#5316=ORIENTED_EDGE('',*,*,#3705,.T.);
#5317=ORIENTED_EDGE('',*,*,#3793,.F.);
#5318=ORIENTED_EDGE('',*,*,#3880,.F.);
#5319=ORIENTED_EDGE('',*,*,#3877,.F.);
#5320=ORIENTED_EDGE('',*,*,#3894,.F.);
#5321=ORIENTED_EDGE('',*,*,#3785,.F.);
#5322=ORIENTED_EDGE('',*,*,#3721,.T.);
#5323=ORIENTED_EDGE('',*,*,#3734,.T.);
#5324=ORIENTED_EDGE('',*,*,#3885,.F.);
#5325=ORIENTED_EDGE('',*,*,#3893,.F.);
#5326=ORIENTED_EDGE('',*,*,#3878,.F.);
#5327=ORIENTED_EDGE('',*,*,#3887,.F.);
#5328=ORIENTED_EDGE('',*,*,#3695,.T.);
#5329=ORIENTED_EDGE('',*,*,#3691,.T.);
#5330=ORIENTED_EDGE('',*,*,#3688,.T.);
#5331=ORIENTED_EDGE('',*,*,#3686,.T.);
#5332=ORIENTED_EDGE('',*,*,#3684,.T.);
#5333=ORIENTED_EDGE('',*,*,#3681,.T.);
#5334=ORIENTED_EDGE('',*,*,#3890,.F.);
#5335=ORIENTED_EDGE('',*,*,#3787,.F.);
#5336=ORIENTED_EDGE('',*,*,#3895,.F.);
#5337=ORIENTED_EDGE('',*,*,#3892,.F.);
#5338=ORIENTED_EDGE('',*,*,#3888,.F.);
#5339=ORIENTED_EDGE('',*,*,#3789,.F.);
#5340=ORIENTED_EDGE('',*,*,#3891,.F.);
#5341=ORIENTED_EDGE('',*,*,#3884,.F.);
#6585=CYLINDRICAL_SURFACE('',#7378,0.15);
#6586=CYLINDRICAL_SURFACE('',#7381,0.15);
#6587=CYLINDRICAL_SURFACE('',#7383,0.15);
#6588=CYLINDRICAL_SURFACE('',#7385,0.15);
#6589=CYLINDRICAL_SURFACE('',#7388,0.3);
#6590=CYLINDRICAL_SURFACE('',#7393,0.3);
#6591=CYLINDRICAL_SURFACE('',#7398,0.17);
#6592=CYLINDRICAL_SURFACE('',#7400,0.17);
#6593=CYLINDRICAL_SURFACE('',#7424,0.4);
#6594=CYLINDRICAL_SURFACE('',#7426,0.4);
#6595=CYLINDRICAL_SURFACE('',#7448,0.1);
#6596=CYLINDRICAL_SURFACE('',#7452,0.1);
#6597=CYLINDRICAL_SURFACE('',#7466,0.3);
#6598=CYLINDRICAL_SURFACE('',#7471,0.3);
#6777=ADVANCED_FACE('',(#898,#608,#609,#610),#707,.F.);
#6778=ADVANCED_FACE('',(#899),#6585,.F.);
#6779=ADVANCED_FACE('',(#900),#6586,.F.);
#6780=ADVANCED_FACE('',(#901),#6587,.F.);
#6781=ADVANCED_FACE('',(#902),#6588,.F.);
#6782=ADVANCED_FACE('',(#903),#6589,.F.);
#6783=ADVANCED_FACE('',(#904,#611),#708,.F.);
#6784=ADVANCED_FACE('',(#905),#6590,.F.);
#6785=ADVANCED_FACE('',(#906,#612),#709,.F.);
#6786=ADVANCED_FACE('',(#907),#6591,.F.);
#6787=ADVANCED_FACE('',(#908),#6592,.F.);
#6788=ADVANCED_FACE('',(#909),#710,.F.);
#6789=ADVANCED_FACE('',(#910),#711,.F.);
#6790=ADVANCED_FACE('',(#911),#712,.F.);
#6791=ADVANCED_FACE('',(#912),#713,.F.);
#6792=ADVANCED_FACE('',(#913),#714,.F.);
#6793=ADVANCED_FACE('',(#914),#715,.F.);
#6794=ADVANCED_FACE('',(#915),#716,.F.);
#6795=ADVANCED_FACE('',(#916,#613),#717,.F.);
#6796=ADVANCED_FACE('',(#917,#614),#718,.F.);
#6797=ADVANCED_FACE('',(#918),#719,.F.);
#6798=ADVANCED_FACE('',(#919),#720,.F.);
#6799=ADVANCED_FACE('',(#920),#721,.F.);
#6800=ADVANCED_FACE('',(#921),#722,.F.);
#6801=ADVANCED_FACE('',(#922),#723,.F.);
#6802=ADVANCED_FACE('',(#923),#724,.T.);
#6803=ADVANCED_FACE('',(#924),#725,.T.);
#6804=ADVANCED_FACE('',(#925),#726,.T.);
#6805=ADVANCED_FACE('',(#926),#727,.T.);
#6806=ADVANCED_FACE('',(#927),#728,.T.);
#6807=ADVANCED_FACE('',(#928,#615),#729,.F.);
#6808=ADVANCED_FACE('',(#929),#6593,.T.);
#6809=ADVANCED_FACE('',(#930),#6594,.T.);
#6810=ADVANCED_FACE('',(#931),#730,.T.);
#6811=ADVANCED_FACE('',(#932),#91,.T.);
#6812=ADVANCED_FACE('',(#933),#92,.T.);
#6813=ADVANCED_FACE('',(#934),#93,.T.);
#6814=ADVANCED_FACE('',(#935),#94,.T.);
#6815=ADVANCED_FACE('',(#936,#616,#617,#618),#731,.F.);
#6816=ADVANCED_FACE('',(#937),#732,.F.);
#6817=ADVANCED_FACE('',(#938),#95,.T.);
#6818=ADVANCED_FACE('',(#939),#96,.T.);
#6819=ADVANCED_FACE('',(#940),#97,.T.);
#6820=ADVANCED_FACE('',(#941),#733,.T.);
#6821=ADVANCED_FACE('',(#942),#98,.T.);
#6822=ADVANCED_FACE('',(#943),#99,.T.);
#6823=ADVANCED_FACE('',(#944),#734,.F.);
#6824=ADVANCED_FACE('',(#945),#100,.T.);
#6825=ADVANCED_FACE('',(#946),#101,.T.);
#6826=ADVANCED_FACE('',(#947),#735,.T.);
#6827=ADVANCED_FACE('',(#948),#102,.T.);
#6828=ADVANCED_FACE('',(#949),#103,.T.);
#6829=ADVANCED_FACE('',(#950),#104,.T.);
#6830=ADVANCED_FACE('',(#951),#105,.T.);
#6831=ADVANCED_FACE('',(#952),#736,.T.);
#6832=ADVANCED_FACE('',(#953),#106,.T.);
#6833=ADVANCED_FACE('',(#954),#107,.T.);
#6834=ADVANCED_FACE('',(#955),#737,.F.);
#6835=ADVANCED_FACE('',(#956),#108,.T.);
#6836=ADVANCED_FACE('',(#957),#109,.T.);
#6837=ADVANCED_FACE('',(#958),#75,.F.);
#6838=ADVANCED_FACE('',(#959),#76,.F.);
#6839=ADVANCED_FACE('',(#960),#77,.F.);
#6840=ADVANCED_FACE('',(#961),#6595,.F.);
#6841=ADVANCED_FACE('',(#962),#110,.T.);
#6842=ADVANCED_FACE('',(#963),#78,.F.);
#6843=ADVANCED_FACE('',(#964),#6596,.F.);
#6844=ADVANCED_FACE('',(#965),#111,.T.);
#6845=ADVANCED_FACE('',(#966),#112,.T.);
#6846=ADVANCED_FACE('',(#967),#113,.T.);
#6847=ADVANCED_FACE('',(#968),#114,.T.);
#6848=ADVANCED_FACE('',(#969),#738,.T.);
#6849=ADVANCED_FACE('',(#970),#79,.T.);
#6850=ADVANCED_FACE('',(#971),#80,.T.);
#6851=ADVANCED_FACE('',(#972),#81,.T.);
#6852=ADVANCED_FACE('',(#973),#6597,.T.);
#6853=ADVANCED_FACE('',(#974),#115,.F.);
#6854=ADVANCED_FACE('',(#975),#82,.T.);
#6855=ADVANCED_FACE('',(#976),#6598,.T.);
#6856=ADVANCED_FACE('',(#977),#116,.F.);
#6857=ADVANCED_FACE('',(#978),#117,.F.);
#6858=ADVANCED_FACE('',(#979),#118,.F.);
#6859=ADVANCED_FACE('',(#980),#119,.F.);
#6860=ADVANCED_FACE('',(#981),#120,.F.);
#6861=ADVANCED_FACE('',(#982),#121,.F.);
#6862=ADVANCED_FACE('',(#983),#739,.F.);
#6863=ADVANCED_FACE('',(#984,#619,#620,#621,#622,#623,#624),#740,.T.);
#6864=ADVANCED_FACE('',(#985),#122,.F.);
#6865=ADVANCED_FACE('',(#986),#741,.F.);
#7107=CLOSED_SHELL('',(#6777,#6778,#6779,#6780,#6781,#6782,#6783,#6784,
#6785,#6786,#6787,#6788,#6789,#6790,#6791,#6792,#6793,#6794,#6795,#6796,
#6797,#6798,#6799,#6800,#6801,#6802,#6803,#6804,#6805,#6806,#6807,#6808,
#6809,#6810,#6811,#6812,#6813,#6814,#6815,#6816,#6817,#6818,#6819,#6820,
#6821,#6822,#6823,#6824,#6825,#6826,#6827,#6828,#6829,#6830,#6831,#6832,
#6833,#6834,#6835,#6836,#6837,#6838,#6839,#6840,#6841,#6842,#6843,#6844,
#6845,#6846,#6847,#6848,#6849,#6850,#6851,#6852,#6853,#6854,#6855,#6856,
#6857,#6858,#6859,#6860,#6861,#6862,#6863,#6864,#6865));
#7373=AXIS2_PLACEMENT_3D('',#9721,#8194,#8195);
#7374=AXIS2_PLACEMENT_3D('',#9722,#8196,#8197);
#7375=AXIS2_PLACEMENT_3D('',#9788,#8200,#8201);
#7376=AXIS2_PLACEMENT_3D('',#9790,#8202,#8203);
#7377=AXIS2_PLACEMENT_3D('',#9792,#8204,#8205);
#7378=AXIS2_PLACEMENT_3D('',#9793,#8206,#8207);
#7379=AXIS2_PLACEMENT_3D('',#9795,#8208,#8209);
#7380=AXIS2_PLACEMENT_3D('',#9798,#8211,#8212);
#7381=AXIS2_PLACEMENT_3D('',#9799,#8213,#8214);
#7382=AXIS2_PLACEMENT_3D('',#9801,#8215,#8216);
#7383=AXIS2_PLACEMENT_3D('',#9803,#8218,#8219);
#7384=AXIS2_PLACEMENT_3D('',#9805,#8220,#8221);
#7385=AXIS2_PLACEMENT_3D('',#9807,#8223,#8224);
#7386=AXIS2_PLACEMENT_3D('',#9809,#8225,#8226);
#7387=AXIS2_PLACEMENT_3D('',#9812,#8228,#8229);
#7388=AXIS2_PLACEMENT_3D('',#9813,#8230,#8231);
#7389=AXIS2_PLACEMENT_3D('',#9815,#8232,#8233);
#7390=AXIS2_PLACEMENT_3D('',#9818,#8235,#8236);
#7391=AXIS2_PLACEMENT_3D('',#9819,#8237,#8238);
#7392=AXIS2_PLACEMENT_3D('',#9821,#8239,#8240);
#7393=AXIS2_PLACEMENT_3D('',#9822,#8241,#8242);
#7394=AXIS2_PLACEMENT_3D('',#9824,#8243,#8244);
#7395=AXIS2_PLACEMENT_3D('',#9827,#8246,#8247);
#7396=AXIS2_PLACEMENT_3D('',#9828,#8248,#8249);
#7397=AXIS2_PLACEMENT_3D('',#9830,#8250,#8251);
#7398=AXIS2_PLACEMENT_3D('',#9831,#8252,#8253);
#7399=AXIS2_PLACEMENT_3D('',#9834,#8255,#8256);
#7400=AXIS2_PLACEMENT_3D('',#9835,#8257,#8258);
#7401=AXIS2_PLACEMENT_3D('',#9838,#8260,#8261);
#7402=AXIS2_PLACEMENT_3D('',#9839,#8262,#8263);
#7403=AXIS2_PLACEMENT_3D('',#9848,#8268,#8269);
#7404=AXIS2_PLACEMENT_3D('',#9857,#8274,#8275);
#7405=AXIS2_PLACEMENT_3D('',#9866,#8280,#8281);
#7406=AXIS2_PLACEMENT_3D('',#9875,#8286,#8287);
#7407=AXIS2_PLACEMENT_3D('',#9884,#8292,#8293);
#7408=AXIS2_PLACEMENT_3D('',#9893,#8298,#8299);
#7409=AXIS2_PLACEMENT_3D('',#9902,#8304,#8305);
#7410=AXIS2_PLACEMENT_3D('',#9904,#8306,#8307);
#7411=AXIS2_PLACEMENT_3D('',#9905,#8308,#8309);
#7412=AXIS2_PLACEMENT_3D('',#9907,#8310,#8311);
#7413=AXIS2_PLACEMENT_3D('',#9908,#8312,#8313);
#7414=AXIS2_PLACEMENT_3D('',#9911,#8316,#8317);
#7415=AXIS2_PLACEMENT_3D('',#9914,#8320,#8321);
#7416=AXIS2_PLACEMENT_3D('',#9917,#8324,#8325);
#7417=AXIS2_PLACEMENT_3D('',#9923,#8329,#8330);
#7418=AXIS2_PLACEMENT_3D('',#9929,#8334,#8335);
#7419=AXIS2_PLACEMENT_3D('',#10006,#8338,#8339);
#7420=AXIS2_PLACEMENT_3D('',#10084,#8343,#8344);
#7421=AXIS2_PLACEMENT_3D('',#10162,#8348,#8349);
#7422=AXIS2_PLACEMENT_3D('',#10237,#8352,#8353);
#7423=AXIS2_PLACEMENT_3D('',#10253,#8357,#8358);
#7424=AXIS2_PLACEMENT_3D('',#10631,#8370,#8371);
#7425=AXIS2_PLACEMENT_3D('',#10633,#8372,#8373);
#7426=AXIS2_PLACEMENT_3D('',#10635,#8375,#8376);
#7427=AXIS2_PLACEMENT_3D('',#10637,#8378,#8379);
#7428=AXIS2_PLACEMENT_3D('',#10805,#8381,#8382);
#7429=AXIS2_PLACEMENT_3D('',#10806,#8383,#8384);
#7430=AXIS2_PLACEMENT_3D('',#10811,#8385,#8386);
#7431=AXIS2_PLACEMENT_3D('',#10883,#8388,#8389);
#7432=AXIS2_PLACEMENT_3D('',#11001,#8391,#8392);
#7433=AXIS2_PLACEMENT_3D('',#11046,#8393,#8394);
#7434=AXIS2_PLACEMENT_3D('',#11197,#8395,#8396);
#7435=AXIS2_PLACEMENT_3D('',#11317,#8398,#8399);
#7436=AXIS2_PLACEMENT_3D('',#11322,#8400,#8401);
#7437=AXIS2_PLACEMENT_3D('',#11374,#8403,#8404);
#7438=AXIS2_PLACEMENT_3D('',#11375,#8405,#8406);
#7439=AXIS2_PLACEMENT_3D('',#11376,#8407,#8408);
#7440=AXIS2_PLACEMENT_3D('',#11377,#8409,#8410);
#7441=AXIS2_PLACEMENT_3D('',#11378,#8411,#8412);
#7442=AXIS2_PLACEMENT_3D('',#11379,#8413,#8414);
#7443=AXIS2_PLACEMENT_3D('',#11381,#8415,#8416);
#7444=AXIS2_PLACEMENT_3D('',#11382,#8417,#8418);
#7445=AXIS2_PLACEMENT_3D('',#11383,#8419,#8420);
#7446=AXIS2_PLACEMENT_3D('',#11384,#8421,#8422);
#7447=AXIS2_PLACEMENT_3D('',#11385,#8423,#8424);
#7448=AXIS2_PLACEMENT_3D('',#11386,#8425,#8426);
#7449=AXIS2_PLACEMENT_3D('',#11407,#8427,#8428);
#7450=AXIS2_PLACEMENT_3D('',#11409,#8429,#8430);
#7451=AXIS2_PLACEMENT_3D('',#11410,#8431,#8432);
#7452=AXIS2_PLACEMENT_3D('',#11411,#8433,#8434);
#7453=AXIS2_PLACEMENT_3D('',#11509,#8436,#8437);
#7454=AXIS2_PLACEMENT_3D('',#11510,#8438,#8439);
#7455=AXIS2_PLACEMENT_3D('',#11513,#8440,#8441);
#7456=AXIS2_PLACEMENT_3D('',#11515,#8442,#8443);
#7457=AXIS2_PLACEMENT_3D('',#11516,#8444,#8445);
#7458=AXIS2_PLACEMENT_3D('',#11517,#8446,#8447);
#7459=AXIS2_PLACEMENT_3D('',#11520,#8448,#8449);
#7460=AXIS2_PLACEMENT_3D('',#11522,#8450,#8451);
#7461=AXIS2_PLACEMENT_3D('',#11523,#8452,#8453);
#7462=AXIS2_PLACEMENT_3D('',#11524,#8454,#8455);
#7463=AXIS2_PLACEMENT_3D('',#11527,#8456,#8457);
#7464=AXIS2_PLACEMENT_3D('',#11529,#8458,#8459);
#7465=AXIS2_PLACEMENT_3D('',#11530,#8460,#8461);
#7466=AXIS2_PLACEMENT_3D('',#11531,#8462,#8463);
#7467=AXIS2_PLACEMENT_3D('',#11562,#8466,#8467);
#7468=AXIS2_PLACEMENT_3D('',#11565,#8468,#8469);
#7469=AXIS2_PLACEMENT_3D('',#11567,#8470,#8471);
#7470=AXIS2_PLACEMENT_3D('',#11568,#8472,#8473);
#7471=AXIS2_PLACEMENT_3D('',#11569,#8474,#8475);
#7472=AXIS2_PLACEMENT_3D('',#11750,#8478,#8479);
#7473=AXIS2_PLACEMENT_3D('',#11751,#8480,#8481);
#7474=AXIS2_PLACEMENT_3D('',#11768,#8482,#8483);
#8194=DIRECTION('axis',(0.,0.,1.));
#8195=DIRECTION('refdir',(1.,0.,0.));
#8196=DIRECTION('center_axis',(-9.61618982193066E-33,1.03600583455278E-18,
1.));
#8197=DIRECTION('ref_axis',(1.,0.,9.61618982193066E-33));
#8198=DIRECTION('',(0.,-1.,1.03600583455278E-18));
#8199=DIRECTION('',(0.,1.,-1.03600583455278E-18));
#8200=DIRECTION('center_axis',(-9.61618982193066E-33,1.03600583455278E-18,
1.));
#8201=DIRECTION('ref_axis',(1.,0.,0.));
#8202=DIRECTION('center_axis',(-9.61618982193066E-33,1.03600583455278E-18,
1.));
#8203=DIRECTION('ref_axis',(1.,0.,0.));
#8204=DIRECTION('center_axis',(-9.61618982193066E-33,1.03600583455278E-18,
1.));
#8205=DIRECTION('ref_axis',(1.,0.,0.));
#8206=DIRECTION('center_axis',(0.,0.,-1.));
#8207=DIRECTION('ref_axis',(1.,0.,0.));
#8208=DIRECTION('center_axis',(9.61618982193066E-33,-1.03600583455278E-18,
-1.));
#8209=DIRECTION('ref_axis',(1.,0.,0.));
#8210=DIRECTION('',(0.,0.,-1.));
#8211=DIRECTION('center_axis',(-9.61618982193066E-33,1.03600583455278E-18,
1.));
#8212=DIRECTION('ref_axis',(1.,0.,0.));
#8213=DIRECTION('center_axis',(0.,0.,-1.));
#8214=DIRECTION('ref_axis',(1.,0.,0.));
#8215=DIRECTION('center_axis',(9.61618982193066E-33,-1.03600583455278E-18,
-1.));
#8216=DIRECTION('ref_axis',(1.,0.,0.));
#8217=DIRECTION('',(0.,0.,-1.));
#8218=DIRECTION('center_axis',(0.,0.,-1.));
#8219=DIRECTION('ref_axis',(1.,0.,0.));
#8220=DIRECTION('center_axis',(9.61618982193066E-33,-1.03600583455278E-18,
-1.));
#8221=DIRECTION('ref_axis',(1.,0.,0.));
#8222=DIRECTION('',(0.,0.,-1.));
#8223=DIRECTION('center_axis',(0.,0.,-1.));
#8224=DIRECTION('ref_axis',(1.,0.,0.));
#8225=DIRECTION('center_axis',(9.61618982193066E-33,-1.03600583455278E-18,
-1.));
#8226=DIRECTION('ref_axis',(1.,0.,0.));
#8227=DIRECTION('',(0.,0.,-1.));
#8228=DIRECTION('center_axis',(-9.61618982193066E-33,1.03600583455278E-18,
1.));
#8229=DIRECTION('ref_axis',(1.,0.,0.));
#8230=DIRECTION('center_axis',(0.,0.,-1.));
#8231=DIRECTION('ref_axis',(1.,0.,0.));
#8232=DIRECTION('center_axis',(9.61618982193066E-33,-1.03600583455278E-18,
-1.));
#8233=DIRECTION('ref_axis',(1.,0.,0.));
#8234=DIRECTION('',(0.,0.,-1.));
#8235=DIRECTION('center_axis',(0.,0.,-1.));
#8236=DIRECTION('ref_axis',(1.,0.,0.));
#8237=DIRECTION('center_axis',(0.,0.,-1.));
#8238=DIRECTION('ref_axis',(1.,0.,0.));
#8239=DIRECTION('center_axis',(0.,0.,1.));
#8240=DIRECTION('ref_axis',(1.,0.,0.));
#8241=DIRECTION('center_axis',(0.,0.,-1.));
#8242=DIRECTION('ref_axis',(1.,0.,0.));
#8243=DIRECTION('center_axis',(9.61618982193066E-33,-1.03600583455278E-18,
-1.));
#8244=DIRECTION('ref_axis',(1.,0.,0.));
#8245=DIRECTION('',(0.,0.,-1.));
#8246=DIRECTION('center_axis',(0.,0.,-1.));
#8247=DIRECTION('ref_axis',(1.,0.,0.));
#8248=DIRECTION('center_axis',(0.,0.,-1.));
#8249=DIRECTION('ref_axis',(1.,0.,0.));
#8250=DIRECTION('center_axis',(0.,0.,1.));
#8251=DIRECTION('ref_axis',(1.,0.,0.));
#8252=DIRECTION('center_axis',(0.,0.,-1.));
#8253=DIRECTION('ref_axis',(1.,0.,0.));
#8254=DIRECTION('',(0.,0.,-1.));
#8255=DIRECTION('center_axis',(0.,0.,1.));
#8256=DIRECTION('ref_axis',(1.,0.,0.));
#8257=DIRECTION('center_axis',(0.,0.,-1.));
#8258=DIRECTION('ref_axis',(1.,0.,0.));
#8259=DIRECTION('',(0.,0.,-1.));
#8260=DIRECTION('center_axis',(0.,0.,1.));
#8261=DIRECTION('ref_axis',(1.,0.,0.));
#8262=DIRECTION('center_axis',(0.,-1.,0.));
#8263=DIRECTION('ref_axis',(-1.,0.,0.));
#8264=DIRECTION('',(0.0523359562429438,0.,0.998629534754574));
#8265=DIRECTION('',(1.,0.,0.));
#8266=DIRECTION('',(-0.0523359562429438,0.,-0.998629534754574));
#8267=DIRECTION('',(1.,0.,0.));
#8268=DIRECTION('center_axis',(0.,-1.,0.));
#8269=DIRECTION('ref_axis',(-1.,0.,0.));
#8270=DIRECTION('',(0.,0.,-1.));
#8271=DIRECTION('',(1.,0.,0.));
#8272=DIRECTION('',(0.,0.,1.));
#8273=DIRECTION('',(1.,0.,0.));
#8274=DIRECTION('center_axis',(0.,-1.,0.));
#8275=DIRECTION('ref_axis',(-1.,0.,0.));
#8276=DIRECTION('',(0.,0.,-1.));
#8277=DIRECTION('',(1.,0.,0.));
#8278=DIRECTION('',(0.,0.,1.));
#8279=DIRECTION('',(1.,0.,0.));
#8280=DIRECTION('center_axis',(0.,-1.,0.));
#8281=DIRECTION('ref_axis',(-1.,0.,0.));
#8282=DIRECTION('',(0.,0.,-1.));
#8283=DIRECTION('',(1.,0.,0.));
#8284=DIRECTION('',(0.,0.,1.));
#8285=DIRECTION('',(1.,0.,0.));
#8286=DIRECTION('center_axis',(0.,1.,0.));
#8287=DIRECTION('ref_axis',(1.,0.,0.));
#8288=DIRECTION('',(-0.0523359562429438,0.,-0.998629534754574));
#8289=DIRECTION('',(-1.,0.,0.));
#8290=DIRECTION('',(0.0523359562429438,0.,0.998629534754574));
#8291=DIRECTION('',(-1.,0.,0.));
#8292=DIRECTION('center_axis',(0.,1.,0.));
#8293=DIRECTION('ref_axis',(1.,0.,0.));
#8294=DIRECTION('',(0.,0.,1.));
#8295=DIRECTION('',(-1.,0.,0.));
#8296=DIRECTION('',(0.,0.,-1.));
#8297=DIRECTION('',(-1.,0.,0.));
#8298=DIRECTION('center_axis',(0.,1.,0.));
#8299=DIRECTION('ref_axis',(1.,0.,0.));
#8300=DIRECTION('',(0.,0.,1.));
#8301=DIRECTION('',(-1.,0.,0.));
#8302=DIRECTION('',(0.,0.,-1.));
#8303=DIRECTION('',(-1.,0.,0.));
#8304=DIRECTION('center_axis',(0.,0.,1.));
#8305=DIRECTION('ref_axis',(1.,0.,0.));
#8306=DIRECTION('center_axis',(0.,0.,1.));
#8307=DIRECTION('ref_axis',(1.,0.,0.));
#8308=DIRECTION('center_axis',(0.,0.,1.));
#8309=DIRECTION('ref_axis',(1.,0.,0.));
#8310=DIRECTION('center_axis',(0.,0.,1.));
#8311=DIRECTION('ref_axis',(1.,0.,0.));
#8312=DIRECTION('center_axis',(0.,0.,1.));
#8313=DIRECTION('ref_axis',(1.,0.,0.));
#8314=DIRECTION('',(0.,1.,0.));
#8315=DIRECTION('',(0.,-1.,0.));
#8316=DIRECTION('center_axis',(0.,0.,1.));
#8317=DIRECTION('ref_axis',(1.,0.,0.));
#8318=DIRECTION('',(0.,-1.,0.));
#8319=DIRECTION('',(0.,1.,0.));
#8320=DIRECTION('center_axis',(0.,0.,1.));
#8321=DIRECTION('ref_axis',(1.,0.,0.));
#8322=DIRECTION('',(0.,-1.,0.));
#8323=DIRECTION('',(0.,1.,0.));
#8324=DIRECTION('center_axis',(0.,0.,1.));
#8325=DIRECTION('ref_axis',(1.,0.,0.));
#8326=DIRECTION('',(0.,-1.,0.));
#8327=DIRECTION('',(-1.,0.,0.));
#8328=DIRECTION('',(0.,1.,0.));
#8329=DIRECTION('center_axis',(0.,1.,0.));
#8330=DIRECTION('ref_axis',(1.,0.,0.));
#8331=DIRECTION('',(0.,0.,1.));
#8332=DIRECTION('',(-1.,0.,0.));
#8333=DIRECTION('',(0.,0.,-1.));
#8334=DIRECTION('center_axis',(-1.,0.,0.));
#8335=DIRECTION('ref_axis',(0.,-1.,0.));
#8336=DIRECTION('',(0.,-1.,0.));
#8337=DIRECTION('',(0.,-1.,1.03600583455278E-18));
#8338=DIRECTION('center_axis',(1.,0.,0.));
#8339=DIRECTION('ref_axis',(0.,1.,0.));
#8340=DIRECTION('',(0.,1.,0.));
#8341=DIRECTION('',(0.,1.,-1.03600583455278E-18));
#8342=DIRECTION('',(0.,1.,0.));
#8343=DIRECTION('center_axis',(1.,0.,0.));
#8344=DIRECTION('ref_axis',(0.,1.,0.));
#8345=DIRECTION('',(0.,1.,0.));
#8346=DIRECTION('',(0.,1.,-1.03600583455278E-18));
#8347=DIRECTION('',(0.,1.,0.));
#8348=DIRECTION('center_axis',(1.,0.,0.));
#8349=DIRECTION('ref_axis',(0.,1.,0.));
#8350=DIRECTION('',(0.,1.,0.));
#8351=DIRECTION('',(0.,1.,0.));
#8352=DIRECTION('center_axis',(0.998629534754574,0.,-0.0523359562429438));
#8353=DIRECTION('ref_axis',(-0.0523359562429438,0.,-0.998629534754574));
#8354=DIRECTION('',(0.,-1.,0.));
#8355=DIRECTION('',(5.42947651131849E-20,-1.,1.03600583455278E-18));
#8356=DIRECTION('',(0.,-1.,0.));
#8357=DIRECTION('center_axis',(0.,0.,1.));
#8358=DIRECTION('ref_axis',(1.,0.,0.));
#8359=DIRECTION('',(0.,-1.,0.));
#8360=DIRECTION('',(0.,-1.,0.));
#8361=DIRECTION('',(0.,-1.,0.));
#8362=DIRECTION('',(0.,1.,0.));
#8363=DIRECTION('',(0.,-1.,0.));
#8364=DIRECTION('',(0.,1.,0.));
#8365=DIRECTION('',(0.,-1.,0.));
#8366=DIRECTION('',(0.,-1.,0.));
#8367=DIRECTION('',(0.,-1.,0.));
#8368=DIRECTION('',(0.,1.,0.));
#8369=DIRECTION('',(0.,1.,0.));
#8370=DIRECTION('center_axis',(0.,0.,1.));
#8371=DIRECTION('ref_axis',(1.,0.,0.));
#8372=DIRECTION('center_axis',(-9.61618982193066E-33,1.03600583455278E-18,
1.));
#8373=DIRECTION('ref_axis',(1.,0.,0.));
#8374=DIRECTION('',(0.,0.,-1.));
#8375=DIRECTION('center_axis',(0.,0.,1.));
#8376=DIRECTION('ref_axis',(1.,0.,0.));
#8377=DIRECTION('',(0.,0.,-1.));
#8378=DIRECTION('center_axis',(1.,0.,0.));
#8379=DIRECTION('ref_axis',(0.,1.,0.));
#8380=DIRECTION('',(0.,1.,-1.03600583455278E-18));
#8381=DIRECTION('center_axis',(0.994044372876412,-0.108976074221552,-1.1933167131821E-14));
#8382=DIRECTION('ref_axis',(-0.108857570442347,-0.992963419871597,0.0466226999892957));
#8383=DIRECTION('center_axis',(-9.61618982193066E-33,1.03600583455278E-18,
1.));
#8384=DIRECTION('ref_axis',(1.,0.,9.61618982193066E-33));
#8385=DIRECTION('center_axis',(-9.61618982193066E-33,1.03600583455278E-18,
1.));
#8386=DIRECTION('ref_axis',(1.,0.,9.61618982193066E-33));
#8387=DIRECTION('',(-5.42947651131849E-20,-1.,1.03600583455278E-18));
#8388=DIRECTION('center_axis',(-1.,0.,0.));
#8389=DIRECTION('ref_axis',(0.,-1.,0.));
#8390=DIRECTION('',(0.,-1.,1.03600583455278E-18));
#8391=DIRECTION('center_axis',(-9.61618982193066E-33,1.03600583455278E-18,
1.));
#8392=DIRECTION('ref_axis',(1.,0.,9.61618982193066E-33));
#8393=DIRECTION('center_axis',(-1.,0.,0.));
#8394=DIRECTION('ref_axis',(0.,-1.,0.));
#8395=DIRECTION('center_axis',(-1.,0.,0.));
#8396=DIRECTION('ref_axis',(0.,-1.,0.));
#8397=DIRECTION('',(0.,-1.,1.03600583455278E-18));
#8398=DIRECTION('center_axis',(-0.999738255753194,0.0228783737088345,0.));
#8399=DIRECTION('ref_axis',(0.,0.,1.));
#8400=DIRECTION('center_axis',(-9.61618982193066E-33,1.03600583455278E-18,
1.));
#8401=DIRECTION('ref_axis',(1.,0.,9.61618982193066E-33));
#8402=DIRECTION('',(-5.42947651131849E-20,1.,-1.03600583455278E-18));
#8403=DIRECTION('center_axis',(-0.999738255790058,-0.0228783720979604,1.69987959829136E-9));
#8404=DIRECTION('ref_axis',(-0.022845652001536,0.998308458201847,0.0534630570326489));
#8405=DIRECTION('center_axis',(-0.375013085256251,-0.833398400631247,0.405970801550885));
#8406=DIRECTION('ref_axis',(-0.565498005067694,0.552672693214782,0.612180447612612));
#8407=DIRECTION('center_axis',(-7.78474640228738E-11,1.,0.));
#8408=DIRECTION('ref_axis',(0.,0.,1.));
#8409=DIRECTION('center_axis',(0.0522645732252412,-0.0522112666801462,0.997267465636596));
#8410=DIRECTION('ref_axis',(-0.998629534754574,0.,0.0523359562429445));
#8411=DIRECTION('center_axis',(0.361627795167438,-0.818371417997736,0.44664701943113));
#8412=DIRECTION('ref_axis',(0.514966362801186,0.574689674697898,0.636035708886648));
#8413=DIRECTION('center_axis',(0.994044372876412,0.108976074221546,-5.96658356591051E-15));
#8414=DIRECTION('ref_axis',(5.9211894646675E-15,7.40148683083438E-16,1.));
#8415=DIRECTION('center_axis',(-0.052263633556273,-0.0525535553916586,0.997249535684621));
#8416=DIRECTION('ref_axis',(-0.108857570442347,0.992963419871597,0.0466226999892949));
#8417=DIRECTION('center_axis',(0.,1.,0.));
#8418=DIRECTION('ref_axis',(0.998629534754574,0.,0.0523359562429438));
#8419=DIRECTION('center_axis',(0.375013085403515,-0.833398400816333,-0.405970801034895));
#8420=DIRECTION('ref_axis',(-0.565498005700927,-0.552672692935682,0.612180447279637));
#8421=DIRECTION('center_axis',(0.0522645732252408,0.0522112666801459,0.997267465636596));
#8422=DIRECTION('ref_axis',(-0.0228456520015352,-0.998308458201847,0.0534630570326489));
#8423=DIRECTION('center_axis',(-4.07418268117644E-12,-1.,-7.77400366303027E-11));
#8424=DIRECTION('ref_axis',(-0.998629534754574,0.,0.0523359562429438));
#8425=DIRECTION('center_axis',(-5.42947651131849E-20,1.,-1.03600583455278E-18));
#8426=DIRECTION('ref_axis',(-0.688354575693754,0.,0.725374371012288));
#8427=DIRECTION('center_axis',(-0.361627795167436,-0.818371417997736,-0.446647019431131));
#8428=DIRECTION('ref_axis',(0.514966362801185,-0.574689674697896,0.636035708886651));
#8429=DIRECTION('center_axis',(-0.0522636335562752,0.0525535553916633,0.99724953568462));
#8430=DIRECTION('ref_axis',(0.998629534754574,0.,0.0523359562429442));
#8431=DIRECTION('center_axis',(0.,-1.,0.));
#8432=DIRECTION('ref_axis',(0.,0.,1.));
#8433=DIRECTION('center_axis',(-5.42947651131849E-20,-1.,1.03600583455278E-18));
#8434=DIRECTION('ref_axis',(0.688354575693754,0.,0.725374371012288));
#8435=DIRECTION('',(5.42947651131849E-20,1.,-1.03600583455278E-18));
#8436=DIRECTION('center_axis',(-0.998629534754574,0.,-0.0523359562429438));
#8437=DIRECTION('ref_axis',(-0.0523359562429438,0.,0.998629534754574));
#8438=DIRECTION('center_axis',(-0.375013085256251,-0.833398400631247,0.405970801550885));
#8439=DIRECTION('ref_axis',(-0.565498005067695,0.552672693214781,0.612180447612612));
#8440=DIRECTION('center_axis',(-7.78474640228738E-11,1.,0.));
#8441=DIRECTION('ref_axis',(0.,0.,1.));
#8442=DIRECTION('center_axis',(-0.999738255790058,-0.0228783720979604,1.69987959829136E-9));
#8443=DIRECTION('ref_axis',(-0.022845652001536,0.998308458201847,0.0534630570326489));
#8444=DIRECTION('center_axis',(0.0522645732252412,-0.0522112666801462,0.997267465636596));
#8445=DIRECTION('ref_axis',(-0.998629534754574,0.,0.0523359562429445));
#8446=DIRECTION('center_axis',(0.361627795167442,-0.818371417997735,0.446647019431129));
#8447=DIRECTION('ref_axis',(0.514966362801186,0.574689674697898,0.636035708886649));
#8448=DIRECTION('center_axis',(0.994044372876412,0.108976074221546,-5.96658356591051E-15));
#8449=DIRECTION('ref_axis',(5.9211894646675E-15,7.40148683083438E-16,1.));
#8450=DIRECTION('center_axis',(0.,1.,0.));
#8451=DIRECTION('ref_axis',(0.998629534754574,0.,0.0523359562429438));
#8452=DIRECTION('center_axis',(-0.052263633556273,-0.0525535553916586,0.997249535684621));
#8453=DIRECTION('ref_axis',(-0.108857570442347,0.992963419871597,0.0466226999892949));
#8454=DIRECTION('center_axis',(0.375013085403515,-0.833398400816333,-0.405970801034895));
#8455=DIRECTION('ref_axis',(-0.565498005700926,-0.552672692935682,0.612180447279637));
#8456=DIRECTION('center_axis',(-0.999738255753194,0.0228783737088345,0.));
#8457=DIRECTION('ref_axis',(0.,0.,1.));
#8458=DIRECTION('center_axis',(-4.07418268117644E-12,-1.,-7.77400366303027E-11));
#8459=DIRECTION('ref_axis',(-0.998629534754574,0.,0.0523359562429438));
#8460=DIRECTION('center_axis',(0.0522645732252408,0.0522112666801459,0.997267465636596));
#8461=DIRECTION('ref_axis',(-0.0228456520015352,-0.998308458201847,0.0534630570326489));
#8462=DIRECTION('center_axis',(-5.42947651131849E-20,1.,-1.03600583455278E-18));
#8463=DIRECTION('ref_axis',(-0.688354575693754,0.,0.725374371012288));
#8464=DIRECTION('',(5.42947651131849E-20,-1.,1.03600583455278E-18));
#8465=DIRECTION('',(-5.42947651131849E-20,1.,-1.03600583455278E-18));
#8466=DIRECTION('center_axis',(-0.361627795167436,-0.818371417997736,-0.446647019431131));
#8467=DIRECTION('ref_axis',(0.51496636280118,-0.574689674697898,0.636035708886653));
#8468=DIRECTION('center_axis',(-0.0522636335562752,0.0525535553916633,0.99724953568462));
#8469=DIRECTION('ref_axis',(0.998629534754574,0.,0.0523359562429441));
#8470=DIRECTION('center_axis',(0.,-1.,0.));
#8471=DIRECTION('ref_axis',(0.,0.,1.));
#8472=DIRECTION('center_axis',(0.994044372876412,-0.108976074221552,-1.1933167131821E-14));
#8473=DIRECTION('ref_axis',(-0.108857570442347,-0.992963419871597,0.0466226999892957));
#8474=DIRECTION('center_axis',(-5.42947651131849E-20,-1.,1.03600583455278E-18));
#8475=DIRECTION('ref_axis',(0.688354575693754,0.,0.725374371012288));
#8476=DIRECTION('',(5.42947651131849E-20,1.,-1.03600583455278E-18));
#8477=DIRECTION('',(-5.42947651131849E-20,-1.,1.03600583455278E-18));
#8478=DIRECTION('center_axis',(0.998629534754574,0.,-0.0523359562429438));
#8479=DIRECTION('ref_axis',(-0.0523359562429438,0.,-0.998629534754574));
#8480=DIRECTION('center_axis',(-9.61618982193066E-33,1.03600583455278E-18,
1.));
#8481=DIRECTION('ref_axis',(1.,0.,9.61618982193066E-33));
#8482=DIRECTION('center_axis',(-0.998629534754574,0.,-0.0523359562429438));
#8483=DIRECTION('ref_axis',(-0.0523359562429438,0.,0.998629534754574));
#9721=CARTESIAN_POINT('',(0.,0.,0.));
#9722=CARTESIAN_POINT('Origin',(6.87409734069396,-2.22251806091942E-16,
0.7));
#9723=CARTESIAN_POINT('',(3.31825992066485,1.2493322588334,0.7));
#9724=CARTESIAN_POINT('',(4.3,1.27917501057225,0.7));
#9725=CARTESIAN_POINT('Ctrl Pts',(3.31826243508713,1.24933270901874,0.7));
#9726=CARTESIAN_POINT('Ctrl Pts',(3.64552542112514,1.25866821321074,0.7));
#9727=CARTESIAN_POINT('Ctrl Pts',(3.97277304530853,1.26856018917077,0.7));
#9728=CARTESIAN_POINT('Ctrl Pts',(4.30000000005992,1.27917501058303,0.7));
#9729=CARTESIAN_POINT('',(4.3,-1.27917501057184,0.7));
#9730=CARTESIAN_POINT('',(4.3,0.742407407407408,0.7));
#9731=CARTESIAN_POINT('',(3.31825992075695,-1.24933225883136,0.7));
#9732=CARTESIAN_POINT('Ctrl Pts',(4.3000000000599,-1.27917501058303,0.7));
#9733=CARTESIAN_POINT('Ctrl Pts',(3.97277304533917,-1.26856018917177,0.7));
#9734=CARTESIAN_POINT('Ctrl Pts',(3.64552542118644,-1.25866821321259,0.7));
#9735=CARTESIAN_POINT('Ctrl Pts',(3.3182624351791,-1.24933270902137,0.7));
#9736=CARTESIAN_POINT('',(3.26759951430388,-1.24789152572578,0.7));
#9737=CARTESIAN_POINT('Ctrl Pts',(3.26760216044043,-1.24789199949781,0.7));
#9738=CARTESIAN_POINT('Ctrl Pts',(3.27154046708102,-1.24840675231115,0.699999999449966));
#9739=CARTESIAN_POINT('Ctrl Pts',(3.27549053112987,-1.2488275353013,0.699997549264952));
#9740=CARTESIAN_POINT('Ctrl Pts',(3.27944900419773,-1.24915404112413,0.699995443099811));
#9741=CARTESIAN_POINT('Ctrl Pts',(3.28202272903949,-1.24936632907779,0.699994073710794));
#9742=CARTESIAN_POINT('Ctrl Pts',(3.28459959180148,-1.24953872742098,0.699992815093061));
#9743=CARTESIAN_POINT('Ctrl Pts',(3.28717866899733,-1.24967118132558,0.699992046536556));
#9744=CARTESIAN_POINT('Ctrl Pts',(3.28888409507617,-1.24975876704947,0.699991538325205));
#9745=CARTESIAN_POINT('Ctrl Pts',(3.29059037034979,-1.2498288805585,0.699991238158591));
#9746=CARTESIAN_POINT('Ctrl Pts',(3.29229723346923,-1.24988151179005,0.69999118215758));
#9747=CARTESIAN_POINT('Ctrl Pts',(3.29393274317941,-1.24993194283473,0.699991128497625));
#9748=CARTESIAN_POINT('Ctrl Pts',(3.29556870469678,-1.24996631998408,0.699991298652463));
#9749=CARTESIAN_POINT('Ctrl Pts',(3.29720488848534,-1.24998463806557,0.699991673963628));
#9750=CARTESIAN_POINT('Ctrl Pts',(3.29943508678369,-1.25000960650399,0.699992185531049));
#9751=CARTESIAN_POINT('Ctrl Pts',(3.30166551218918,-1.25000473681137,0.699993084765318));
#9752=CARTESIAN_POINT('Ctrl Pts',(3.30389557412726,-1.24997002667259,0.699994176731177));
#9753=CARTESIAN_POINT('Ctrl Pts',(3.30868977915254,-1.24989540653807,0.699996524248132));
#9754=CARTESIAN_POINT('Ctrl Pts',(3.31348068594496,-1.24968290539118,0.699999999312134));
#9755=CARTESIAN_POINT('Ctrl Pts',(3.3182624351791,-1.24933270902137,0.7));
#9756=CARTESIAN_POINT('',(1.1,-1.19266190204492,0.7));
#9757=CARTESIAN_POINT('Ctrl Pts',(3.26760216044045,-1.24789199949781,0.7));
#9758=CARTESIAN_POINT('Ctrl Pts',(2.54512260523322,-1.2274084473838,0.7));
#9759=CARTESIAN_POINT('Ctrl Pts',(1.82256951666701,-1.20959509718369,0.7));
#9760=CARTESIAN_POINT('Ctrl Pts',(1.09999999999999,-1.19266190204553,0.7));
#9761=CARTESIAN_POINT('',(1.1,1.19266190204492,0.7));
#9762=CARTESIAN_POINT('',(1.1,-0.696450594095222,0.7));
#9763=CARTESIAN_POINT('',(3.26759952419083,1.24789152650872,0.7));
#9764=CARTESIAN_POINT('Ctrl Pts',(1.09999999999999,1.19266190204553,0.7));
#9765=CARTESIAN_POINT('Ctrl Pts',(1.82256951996781,1.20959509726105,0.7));
#9766=CARTESIAN_POINT('Ctrl Pts',(2.54512261183467,1.22740844754655,0.7));
#9767=CARTESIAN_POINT('Ctrl Pts',(3.26760217034162,1.24789199977852,0.7));
#9768=CARTESIAN_POINT('Ctrl Pts',(3.3182624351791,1.24933270902137,0.7));
#9769=CARTESIAN_POINT('Ctrl Pts',(3.3143012451848,1.2496228108833,0.699999999430174));
#9770=CARTESIAN_POINT('Ctrl Pts',(3.31033365565543,1.24981842655856,0.699997549220164));
#9771=CARTESIAN_POINT('Ctrl Pts',(3.30636302717881,1.24991943948955,0.699995443052606));
#9772=CARTESIAN_POINT('Ctrl Pts',(3.30378139908369,1.24998511620097,0.699994073661998));
#9773=CARTESIAN_POINT('Ctrl Pts',(3.3011989045204,1.25001078941611,0.699992815050698));
#9774=CARTESIAN_POINT('Ctrl Pts',(3.29861646861803,1.2499964568765,0.699992046505716));
#9775=CARTESIAN_POINT('Ctrl Pts',(3.2969088217217,1.24998697942277,0.699991538302026));
#9776=CARTESIAN_POINT('Ctrl Pts',(3.29520131971864,1.24996000972381,0.699991238145114));
#9777=CARTESIAN_POINT('Ctrl Pts',(3.29349422410899,1.24991555258537,0.699991182154076));
#9778=CARTESIAN_POINT('Ctrl Pts',(3.29185849176351,1.24987295392896,0.699991128503682));
#9779=CARTESIAN_POINT('Ctrl Pts',(3.29022322047391,1.2498143016413,0.699991298668259));
#9780=CARTESIAN_POINT('Ctrl Pts',(3.28858863969825,1.2497396036024,0.699991673987721));
#9781=CARTESIAN_POINT('Ctrl Pts',(3.286360626573,1.24963778654105,0.699992185566407));
#9782=CARTESIAN_POINT('Ctrl Pts',(3.28413408201674,1.24950616665997,0.699993084809042));
#9783=CARTESIAN_POINT('Ctrl Pts',(3.2819095957713,1.24934477520901,0.699994176777649));
#9784=CARTESIAN_POINT('Ctrl Pts',(3.27712738077041,1.24899781481787,0.699996524298861));
#9785=CARTESIAN_POINT('Ctrl Pts',(3.27235629258357,1.24851338385513,0.699999999330822));
#9786=CARTESIAN_POINT('Ctrl Pts',(3.26760217026193,1.24789200078152,0.699999999999999));
#9787=CARTESIAN_POINT('',(3.15,1.,0.7));
#9788=CARTESIAN_POINT('Origin',(3.3,1.,0.7));
#9789=CARTESIAN_POINT('',(3.15,-1.,0.7));
#9790=CARTESIAN_POINT('Origin',(3.3,-1.,0.7));
#9791=CARTESIAN_POINT('',(1.6,-4.89858719658941E-17,0.7));
#9792=CARTESIAN_POINT('Origin',(2.,0.,0.7));
#9793=CARTESIAN_POINT('Origin',(9.9,-1.,0.8));
#9794=CARTESIAN_POINT('',(9.75,-1.,0.9));
#9795=CARTESIAN_POINT('Origin',(9.9,-1.,0.9));
#9796=CARTESIAN_POINT('',(9.75,-1.,0.7));
#9797=CARTESIAN_POINT('',(9.75,-1.,0.8));
#9798=CARTESIAN_POINT('Origin',(9.9,-1.,0.7));
#9799=CARTESIAN_POINT('Origin',(3.3,-1.,0.8));
#9800=CARTESIAN_POINT('',(3.15,-1.,0.9));
#9801=CARTESIAN_POINT('Origin',(3.3,-1.,0.9));
#9802=CARTESIAN_POINT('',(3.15,-1.,0.8));
#9803=CARTESIAN_POINT('Origin',(3.3,1.,0.8));
#9804=CARTESIAN_POINT('',(3.15,1.,0.9));
#9805=CARTESIAN_POINT('Origin',(3.3,1.,0.9));
#9806=CARTESIAN_POINT('',(3.15,1.,0.8));
#9807=CARTESIAN_POINT('Origin',(9.9,1.,0.8));
#9808=CARTESIAN_POINT('',(9.75,1.,0.9));
#9809=CARTESIAN_POINT('Origin',(9.9,1.,0.9));
#9810=CARTESIAN_POINT('',(9.75,1.,0.7));
#9811=CARTESIAN_POINT('',(9.75,1.,0.8));
#9812=CARTESIAN_POINT('Origin',(9.9,1.,0.7));
#9813=CARTESIAN_POINT('Origin',(2.,0.,0.75));
#9814=CARTESIAN_POINT('',(1.7,3.67394039744206E-17,0.9));
#9815=CARTESIAN_POINT('Origin',(2.,0.,0.9));
#9816=CARTESIAN_POINT('',(1.7,3.67394039744206E-17,0.6));
#9817=CARTESIAN_POINT('',(1.7,3.67394039744206E-17,0.75));
#9818=CARTESIAN_POINT('Origin',(2.,0.,0.6));
#9819=CARTESIAN_POINT('Origin',(2.,0.,0.6));
#9820=CARTESIAN_POINT('',(1.83,-2.0818995585505E-17,0.6));
#9821=CARTESIAN_POINT('Origin',(2.,0.,0.6));
#9822=CARTESIAN_POINT('Origin',(11.2,0.,0.75));
#9823=CARTESIAN_POINT('',(10.9,3.67394039744206E-17,0.9));
#9824=CARTESIAN_POINT('Origin',(11.2,0.,0.9));
#9825=CARTESIAN_POINT('',(10.9,3.67394039744206E-17,0.6));
#9826=CARTESIAN_POINT('',(10.9,3.67394039744206E-17,0.75));
#9827=CARTESIAN_POINT('Origin',(11.2,0.,0.6));
#9828=CARTESIAN_POINT('Origin',(11.2,0.,0.6));
#9829=CARTESIAN_POINT('',(11.03,-2.0818995585505E-17,0.6));
#9830=CARTESIAN_POINT('Origin',(11.2,0.,0.6));
#9831=CARTESIAN_POINT('Origin',(2.,0.,0.45));
#9832=CARTESIAN_POINT('',(1.83,-2.0818995585505E-17,0.32));
#9833=CARTESIAN_POINT('',(1.83,2.0818995585505E-17,0.45));
#9834=CARTESIAN_POINT('Origin',(2.,0.,0.32));
#9835=CARTESIAN_POINT('Origin',(11.2,0.,0.45));
#9836=CARTESIAN_POINT('',(11.03,-2.0818995585505E-17,0.32));
#9837=CARTESIAN_POINT('',(11.03,2.0818995585505E-17,0.45));
#9838=CARTESIAN_POINT('Origin',(11.2,0.,0.32));
#9839=CARTESIAN_POINT('Origin',(12.4,-0.72,0.32));
#9840=CARTESIAN_POINT('',(0.200274469199584,-0.72,0.));
#9841=CARTESIAN_POINT('',(0.217044958570157,-0.72,0.32));
#9842=CARTESIAN_POINT('',(0.225070308370679,-0.72,0.473132796510599));
#9843=CARTESIAN_POINT('',(0.,-0.72,0.));
#9844=CARTESIAN_POINT('',(9.63649764092939,-0.72,0.));
#9845=CARTESIAN_POINT('',(0.0167704893705732,-0.72,0.32));
#9846=CARTESIAN_POINT('',(0.0253444014197637,-0.72,0.483599987759188));
#9847=CARTESIAN_POINT('',(-0.1,-0.72,0.32));
#9848=CARTESIAN_POINT('Origin',(12.4,-0.72,0.32));
#9849=CARTESIAN_POINT('',(0.9,-0.72,0.32));
#9850=CARTESIAN_POINT('',(0.9,-0.72,0.));
#9851=CARTESIAN_POINT('',(0.9,-0.72,0.16));
#9852=CARTESIAN_POINT('',(1.1,-0.72,0.32));
#9853=CARTESIAN_POINT('',(-0.1,-0.72,0.32));
#9854=CARTESIAN_POINT('',(1.1,-0.72,0.));
#9855=CARTESIAN_POINT('',(1.1,-0.72,0.16));
#9856=CARTESIAN_POINT('',(9.63649764092939,-0.72,0.));
#9857=CARTESIAN_POINT('Origin',(12.4,-0.72,0.32));
#9858=CARTESIAN_POINT('',(4.3,-0.72,0.32));
#9859=CARTESIAN_POINT('',(4.3,-0.72,0.));
#9860=CARTESIAN_POINT('',(4.3,-0.72,0.16));
#9861=CARTESIAN_POINT('',(4.5,-0.72,0.32));
#9862=CARTESIAN_POINT('',(-0.1,-0.72,0.32));
#9863=CARTESIAN_POINT('',(4.5,-0.72,0.));
#9864=CARTESIAN_POINT('',(4.5,-0.72,0.16));
#9865=CARTESIAN_POINT('',(9.63649764092939,-0.72,0.));
#9866=CARTESIAN_POINT('Origin',(12.4,-0.72,0.32));
#9867=CARTESIAN_POINT('',(8.7,-0.72,0.32));
#9868=CARTESIAN_POINT('',(8.7,-0.72,0.));
#9869=CARTESIAN_POINT('',(8.7,-0.72,0.16));
#9870=CARTESIAN_POINT('',(8.9,-0.72,0.32));
#9871=CARTESIAN_POINT('',(-0.1,-0.72,0.32));
#9872=CARTESIAN_POINT('',(8.9,-0.72,0.));
#9873=CARTESIAN_POINT('',(8.9,-0.72,0.16));
#9874=CARTESIAN_POINT('',(9.63649764092939,-0.72,0.));
#9875=CARTESIAN_POINT('Origin',(-0.0999999999999996,0.72,0.32));
#9876=CARTESIAN_POINT('',(0.217044958570158,0.72,0.32));
#9877=CARTESIAN_POINT('',(0.200274469199584,0.72,0.));
#9878=CARTESIAN_POINT('',(0.207951231396534,0.72,0.146481348799182));
#9879=CARTESIAN_POINT('',(0.0167704893705736,0.72,0.32));
#9880=CARTESIAN_POINT('',(12.4,0.72,0.32));
#9881=CARTESIAN_POINT('',(0.,0.72,0.));
#9882=CARTESIAN_POINT('',(0.00822532444561912,0.72,0.156948540047771));
#9883=CARTESIAN_POINT('',(3.38649764092939,0.72,0.));
#9884=CARTESIAN_POINT('Origin',(-0.0999999999999996,0.72,0.32));
#9885=CARTESIAN_POINT('',(0.9,0.72,0.));
#9886=CARTESIAN_POINT('',(0.9,0.72,0.32));
#9887=CARTESIAN_POINT('',(0.9,0.72,0.16));
#9888=CARTESIAN_POINT('',(1.1,0.72,0.));
#9889=CARTESIAN_POINT('',(3.38649764092939,0.72,0.));
#9890=CARTESIAN_POINT('',(1.1,0.72,0.32));
#9891=CARTESIAN_POINT('',(1.1,0.72,0.16));
#9892=CARTESIAN_POINT('',(12.4,0.72,0.32));
#9893=CARTESIAN_POINT('Origin',(-0.0999999999999996,0.72,0.32));
#9894=CARTESIAN_POINT('',(4.3,0.72,0.));
#9895=CARTESIAN_POINT('',(4.3,0.72,0.32));
#9896=CARTESIAN_POINT('',(4.3,0.72,0.16));
#9897=CARTESIAN_POINT('',(4.5,0.72,0.));
#9898=CARTESIAN_POINT('',(3.38649764092939,0.72,0.));
#9899=CARTESIAN_POINT('',(4.5,0.72,0.32));
#9900=CARTESIAN_POINT('',(4.5,0.72,0.16));
#9901=CARTESIAN_POINT('',(12.4,0.72,0.32));
#9902=CARTESIAN_POINT('Origin',(6.15,0.,0.32));
#9903=CARTESIAN_POINT('',(1.6,-4.89858719658941E-17,0.32));
#9904=CARTESIAN_POINT('Origin',(2.,0.,0.32));
#9905=CARTESIAN_POINT('Origin',(6.15,0.,0.32));
#9906=CARTESIAN_POINT('',(10.8,-4.89858719658942E-17,0.32));
#9907=CARTESIAN_POINT('Origin',(11.2,0.,0.32));
#9908=CARTESIAN_POINT('Origin',(6.15,0.,0.32));
#9909=CARTESIAN_POINT('',(0.217044958570157,-0.75,0.32));
#9910=CARTESIAN_POINT('',(0.0167704893705736,-0.75,0.32));
#9911=CARTESIAN_POINT('Origin',(6.15,0.,0.32));
#9912=CARTESIAN_POINT('',(0.9,0.696450594095222,0.32));
#9913=CARTESIAN_POINT('',(1.1,-0.696450594095222,0.32));
#9914=CARTESIAN_POINT('Origin',(6.15,0.,0.32));
#9915=CARTESIAN_POINT('',(4.3,0.742407407407408,0.32));
#9916=CARTESIAN_POINT('',(4.5,-0.742407407407408,0.32));
#9917=CARTESIAN_POINT('Origin',(6.15,0.,0.32));
#9918=CARTESIAN_POINT('',(8.7,0.72,0.32));
#9919=CARTESIAN_POINT('',(8.7,0.844259259259259,0.32));
#9920=CARTESIAN_POINT('',(8.9,0.72,0.32));
#9921=CARTESIAN_POINT('',(12.4,0.72,0.32));
#9922=CARTESIAN_POINT('',(8.9,-0.844259259259259,0.32));
#9923=CARTESIAN_POINT('Origin',(-0.0999999999999996,0.72,0.32));
#9924=CARTESIAN_POINT('',(8.7,0.72,0.));
#9925=CARTESIAN_POINT('',(8.7,0.72,0.16));
#9926=CARTESIAN_POINT('',(8.9,0.72,0.));
#9927=CARTESIAN_POINT('',(3.38649764092939,0.72,0.));
#9928=CARTESIAN_POINT('',(8.9,0.72,0.16));
#9929=CARTESIAN_POINT('Origin',(12.4,1.99376954809806,0.));
#9930=CARTESIAN_POINT('',(12.4,1.91212902562343,0.));
#9931=CARTESIAN_POINT('',(12.4,-1.91212902562343,0.));
#9932=CARTESIAN_POINT('',(12.4,1.99376954809806,0.));
#9933=CARTESIAN_POINT('',(12.4,-1.8833055216247,0.604732563714112));
#9934=CARTESIAN_POINT('Ctrl Pts',(12.4,-1.8833055216247,0.604732563714112));
#9935=CARTESIAN_POINT('Ctrl Pts',(12.4,-1.88809880980762,0.504101072758768));
#9936=CARTESIAN_POINT('Ctrl Pts',(12.4,-1.89289370245628,0.403468941627095));
#9937=CARTESIAN_POINT('Ctrl Pts',(12.4,-1.90250151416087,0.201891903194028));
#9938=CARTESIAN_POINT('Ctrl Pts',(12.4,-1.90731451170285,0.100945553925438));
#9939=CARTESIAN_POINT('Ctrl Pts',(12.4,-1.91212902562343,0.));
#9940=CARTESIAN_POINT('',(12.4,-1.78288409287054,0.7));
#9941=CARTESIAN_POINT('Ctrl Pts',(12.4000000030461,-1.78288409409899,0.7));
#9942=CARTESIAN_POINT('Ctrl Pts',(12.4000000066823,-1.79082830277209,0.699999997040196));
#9943=CARTESIAN_POINT('Ctrl Pts',(12.4000021328137,-1.79871128857748,0.699006690321208));
#9944=CARTESIAN_POINT('Ctrl Pts',(12.4000039827682,-1.8063921320806,0.697119229445379));
#9945=CARTESIAN_POINT('Ctrl Pts',(12.4000049365067,-1.81035196808589,0.69614615460905));
#9946=CARTESIAN_POINT('Ctrl Pts',(12.4000058167808,-1.81425808325963,0.694934510320783));
#9947=CARTESIAN_POINT('Ctrl Pts',(12.400006432968,-1.81808986884151,0.693492707237305));
#9948=CARTESIAN_POINT('Ctrl Pts',(12.4000076352846,-1.82556652433459,0.690679432664999));
#9949=CARTESIAN_POINT('Ctrl Pts',(12.4000076271954,-1.83268048852469,0.687023315130674));
#9950=CARTESIAN_POINT('Ctrl Pts',(12.4000063864816,-1.83928589538344,0.682605693351404));
#9951=CARTESIAN_POINT('Ctrl Pts',(12.4000055969106,-1.84348947395919,0.679794387301037));
#9952=CARTESIAN_POINT('Ctrl Pts',(12.400004329084,-1.84748689691167,0.676673627174617));
#9953=CARTESIAN_POINT('Ctrl Pts',(12.4000032503406,-1.8512341074341,0.673255429390325));
#9954=CARTESIAN_POINT('Ctrl Pts',(12.4000023796213,-1.85425870830395,0.670496394655072));
#9955=CARTESIAN_POINT('Ctrl Pts',(12.4000016297172,-1.85710218072175,0.667559826261508));
#9956=CARTESIAN_POINT('Ctrl Pts',(12.4000016274617,-1.859744520612,0.664455546516084));
#9957=CARTESIAN_POINT('Ctrl Pts',(12.4000016230979,-1.86485672743849,0.658449612092435));
#9958=CARTESIAN_POINT('Ctrl Pts',(12.4000041080363,-1.86921906069885,0.651817317967817));
#9959=CARTESIAN_POINT('Ctrl Pts',(12.40000495371,-1.8727702927896,0.64472299566344));
#9960=CARTESIAN_POINT('Ctrl Pts',(12.4000050555652,-1.8731980125259,0.643868536819953));
#9961=CARTESIAN_POINT('Ctrl Pts',(12.4000051394069,-1.87361391018412,0.643007349425002));
#9962=CARTESIAN_POINT('Ctrl Pts',(12.4000052029357,-1.87401783114888,0.642139703315781));
#9963=CARTESIAN_POINT('Ctrl Pts',(12.4000057294153,-1.87736522853405,0.634949295858174));
#9964=CARTESIAN_POINT('Ctrl Pts',(12.4000043880804,-1.87985460663586,0.627401584261416));
#9965=CARTESIAN_POINT('Ctrl Pts',(12.4000025112034,-1.88143175301701,0.619663949188762));
#9966=CARTESIAN_POINT('Ctrl Pts',(12.4000013193515,-1.88243327046239,0.614750406220363));
#9967=CARTESIAN_POINT('Ctrl Pts',(12.4,-1.88306607129604,0.609759643802656));
#9968=CARTESIAN_POINT('Ctrl Pts',(12.4,-1.8833055216247,0.604732563714112));
#9969=CARTESIAN_POINT('',(12.4,1.78288409287164,0.7));
#9970=CARTESIAN_POINT('',(12.4,0.99688477404903,0.7));
#9971=CARTESIAN_POINT('',(12.4,1.8833055216247,0.604732563714112));
#9972=CARTESIAN_POINT('Ctrl Pts',(12.4,1.8833055216247,0.604732563714112));
#9973=CARTESIAN_POINT('Ctrl Pts',(12.4,1.88292893537322,0.612638709665068));
#9974=CARTESIAN_POINT('Ctrl Pts',(12.4000029905988,1.88158186833012,0.620459457162159));
#9975=CARTESIAN_POINT('Ctrl Pts',(12.400004351969,1.87934739482834,0.62803467841275));
#9976=CARTESIAN_POINT('Ctrl Pts',(12.4000050124983,1.87826324073514,0.631710133556493));
#9977=CARTESIAN_POINT('Ctrl Pts',(12.4000053733669,1.87696936339782,0.63532777623417));
#9978=CARTESIAN_POINT('Ctrl Pts',(12.4000053391329,1.87547104796815,0.638868146717817));
#9979=CARTESIAN_POINT('Ctrl Pts',(12.4000052683671,1.872373843052,0.646186534188034));
#9980=CARTESIAN_POINT('Ctrl Pts',(12.4000032465668,1.86844110215533,0.653093304890266));
#9981=CARTESIAN_POINT('Ctrl Pts',(12.4000021327941,1.86374151467895,0.659427433016556));
#9982=CARTESIAN_POINT('Ctrl Pts',(12.4000018304335,1.86246569800928,0.66114698527342));
#9983=CARTESIAN_POINT('Ctrl Pts',(12.4000016226794,1.86113309763036,0.662824214875179));
#9984=CARTESIAN_POINT('Ctrl Pts',(12.400001625255,1.85974452038344,0.664455546516227));
#9985=CARTESIAN_POINT('Ctrl Pts',(12.4000016287814,1.85784336180007,0.666689070188443));
#9986=CARTESIAN_POINT('Ctrl Pts',(12.400002024929,1.85583728779192,0.668836587948716));
#9987=CARTESIAN_POINT('Ctrl Pts',(12.4000025639666,1.85373364862045,0.670894373083513));
#9988=CARTESIAN_POINT('Ctrl Pts',(12.400004021536,1.84804536272624,0.676458668669153));
#9989=CARTESIAN_POINT('Ctrl Pts',(12.4000062945443,1.84171268252251,0.681305055194542));
#9990=CARTESIAN_POINT('Ctrl Pts',(12.4000070319583,1.83490078417639,0.685381489016216));
#9991=CARTESIAN_POINT('Ctrl Pts',(12.4000075068619,1.8305138392177,0.688006761722114));
#9992=CARTESIAN_POINT('Ctrl Pts',(12.4000074483741,1.82592714021755,0.69031203082117));
#9993=CARTESIAN_POINT('Ctrl Pts',(12.4000068708525,1.82117863971551,0.692273867243687));
#9994=CARTESIAN_POINT('Ctrl Pts',(12.4000059767178,1.81382688138917,0.695311236040001));
#9995=CARTESIAN_POINT('Ctrl Pts',(12.4000038254996,1.80617119073902,0.697493343451155));
#9996=CARTESIAN_POINT('Ctrl Pts',(12.4000020685374,1.7983596509798,0.698751345219246));
#9997=CARTESIAN_POINT('Ctrl Pts',(12.4000009204513,1.79325520389048,0.699573385900268));
#9998=CARTESIAN_POINT('Ctrl Pts',(12.400000005426,1.78808359082883,0.699999998062804));
#9999=CARTESIAN_POINT('Ctrl Pts',(12.4000000030461,1.78288409409899,0.7));
#10000=CARTESIAN_POINT('Ctrl Pts',(12.4,1.91212902562343,0.));
#10001=CARTESIAN_POINT('Ctrl Pts',(12.4,1.90731404243129,0.1009553931071));
#10002=CARTESIAN_POINT('Ctrl Pts',(12.4,1.9025005759122,0.201911581737034));
#10003=CARTESIAN_POINT('Ctrl Pts',(12.4,1.89289276481806,0.403488620176902));
#10004=CARTESIAN_POINT('Ctrl Pts',(12.4,1.88809834114759,0.504110911924693));
#10005=CARTESIAN_POINT('Ctrl Pts',(12.4,1.8833055216247,0.604732563714112));
#10006=CARTESIAN_POINT('Origin',(8.9,-1.68851851851852,0.));
#10007=CARTESIAN_POINT('',(8.9,1.62420669932031,0.));
#10008=CARTESIAN_POINT('',(8.9,-1.68851851851852,0.));
#10009=CARTESIAN_POINT('',(8.9,1.59320117118329,0.605106081470792));
#10010=CARTESIAN_POINT('Ctrl Pts',(8.9,1.59320117118329,0.605106081470792));
#10011=CARTESIAN_POINT('Ctrl Pts',(8.9,1.59837103562161,0.504197738990529));
#10012=CARTESIAN_POINT('Ctrl Pts',(8.9,1.60354126123154,0.403288838380538));
#10013=CARTESIAN_POINT('Ctrl Pts',(8.9,1.61387642009944,0.201587196710533));
#10014=CARTESIAN_POINT('Ctrl Pts',(8.9,1.61904141157348,0.100793304842659));
#10015=CARTESIAN_POINT('Ctrl Pts',(8.9,1.62420669932031,0.));
#10016=CARTESIAN_POINT('',(8.9,1.49312521822106,0.7));
#10017=CARTESIAN_POINT('Ctrl Pts',(8.9,1.49312521822106,0.7));
#10018=CARTESIAN_POINT('Ctrl Pts',(8.9,1.50104136823484,0.7));
#10019=CARTESIAN_POINT('Ctrl Pts',(8.90000131173634,1.50889623314995,0.699007530025307));
#10020=CARTESIAN_POINT('Ctrl Pts',(8.90000245364087,1.51654949575132,0.697121675771258));
#10021=CARTESIAN_POINT('Ctrl Pts',(8.9000030153269,1.52031402289636,0.696194051841344));
#10022=CARTESIAN_POINT('Ctrl Pts',(8.90000353645954,1.52402976767023,0.695049421358208));
#10023=CARTESIAN_POINT('Ctrl Pts',(8.90000391188735,1.52767894577544,0.693695149285802));
#10024=CARTESIAN_POINT('Ctrl Pts',(8.90000468147812,1.53515940869299,0.690919022244083));
#10025=CARTESIAN_POINT('Ctrl Pts',(8.90000470661952,1.54227958804117,0.687295426711095));
#10026=CARTESIAN_POINT('Ctrl Pts',(8.9000039635008,1.54889410374269,0.682907715777054));
#10027=CARTESIAN_POINT('Ctrl Pts',(8.90000349228854,1.55308837416723,0.680125464281631));
#10028=CARTESIAN_POINT('Ctrl Pts',(8.90000272405863,1.55707914411963,0.677034908766328));
#10029=CARTESIAN_POINT('Ctrl Pts',(8.90000205379677,1.56082314136721,0.673648333128258));
#10030=CARTESIAN_POINT('Ctrl Pts',(8.90000149471997,1.56394607304962,0.670823532879853));
#10031=CARTESIAN_POINT('Ctrl Pts',(8.90000100172653,1.56687805273397,0.667809941545923));
#10032=CARTESIAN_POINT('Ctrl Pts',(8.90000100003,1.56959740049228,0.664618488856983));
#10033=CARTESIAN_POINT('Ctrl Pts',(8.90000099684156,1.57470809805256,0.658620525035968));
#10034=CARTESIAN_POINT('Ctrl Pts',(8.90000253934467,1.57907071782202,0.651995745956818));
#10035=CARTESIAN_POINT('Ctrl Pts',(8.90000305932469,1.58262507990443,0.644909256877938));
#10036=CARTESIAN_POINT('Ctrl Pts',(8.90000311559331,1.58300970826793,0.644142406277414));
#10037=CARTESIAN_POINT('Ctrl Pts',(8.9000031627798,1.58338482682255,0.643370127200485));
#10038=CARTESIAN_POINT('Ctrl Pts',(8.90000319981124,1.58375032531468,0.642592615892991));
#10039=CARTESIAN_POINT('Ctrl Pts',(8.90000354178946,1.58712563340961,0.635412448897651));
#10040=CARTESIAN_POINT('Ctrl Pts',(8.90000272882427,1.58964525157545,0.627871187463612));
#10041=CARTESIAN_POINT('Ctrl Pts',(8.90000156924769,1.59125549206429,0.620136848214628));
#10042=CARTESIAN_POINT('Ctrl Pts',(8.90000082792478,1.59228492658837,0.615192247765769));
#10043=CARTESIAN_POINT('Ctrl Pts',(8.89999999997262,1.59294182914154,0.610168076493048));
#10044=CARTESIAN_POINT('Ctrl Pts',(8.9000000009702,1.5932011715731,0.605106081469384));
#10045=CARTESIAN_POINT('',(8.9,-1.49312521822001,0.7));
#10046=CARTESIAN_POINT('',(8.9,-0.844259259259259,0.7));
#10047=CARTESIAN_POINT('',(8.9,-1.59320117118329,0.605106081470792));
#10048=CARTESIAN_POINT('Ctrl Pts',(8.90000000097019,-1.5932011715731,0.605106081469384));
#10049=CARTESIAN_POINT('Ctrl Pts',(8.89999999941083,-1.59279578158415,0.613018716877257));
#10050=CARTESIAN_POINT('Ctrl Pts',(8.90000185372291,-1.59142151714118,0.620841302874248));
#10051=CARTESIAN_POINT('Ctrl Pts',(8.90000269095591,-1.58916270068609,0.628413601005994));
#10052=CARTESIAN_POINT('Ctrl Pts',(8.90000316003867,-1.58789713677684,0.632656188846207));
#10053=CARTESIAN_POINT('Ctrl Pts',(8.90000337414869,-1.58635289833986,0.636820251299613));
#10054=CARTESIAN_POINT('Ctrl Pts',(8.90000326408749,-1.58453800492682,0.640875626603871));
#10055=CARTESIAN_POINT('Ctrl Pts',(8.9000030675631,-1.58129734600662,0.648116871770122));
#10056=CARTESIAN_POINT('Ctrl Pts',(8.90000169351568,-1.5772322800227,0.654932667693845));
#10057=CARTESIAN_POINT('Ctrl Pts',(8.90000116172667,-1.57240747726376,0.66116027211862));
#10058=CARTESIAN_POINT('Ctrl Pts',(8.90000106146602,-1.57149783490479,0.662334391157823));
#10059=CARTESIAN_POINT('Ctrl Pts',(8.90000099955281,-1.57056105641498,0.663487533005214));
#10060=CARTESIAN_POINT('Ctrl Pts',(8.90000100072893,-1.56959740053727,0.664618488856962));
#10061=CARTESIAN_POINT('Ctrl Pts',(8.9000010030487,-1.56769671285427,0.666849154291726));
#10062=CARTESIAN_POINT('Ctrl Pts',(8.90000124864079,-1.56569149899762,0.668993559652069));
#10063=CARTESIAN_POINT('Ctrl Pts',(8.90000158179872,-1.56358911460694,0.671047966011734));
#10064=CARTESIAN_POINT('Ctrl Pts',(8.90000248280001,-1.55790336961918,0.676603957919834));
#10065=CARTESIAN_POINT('Ctrl Pts',(8.90000387848177,-1.55157399841983,0.681441805123218));
#10066=CARTESIAN_POINT('Ctrl Pts',(8.90000432886686,-1.54476515293017,0.68550782533293));
#10067=CARTESIAN_POINT('Ctrl Pts',(8.9000046162921,-1.54041990676133,0.688102664467623));
#10068=CARTESIAN_POINT('Ctrl Pts',(8.90000458123012,-1.53587841548674,0.69038248607508));
#10069=CARTESIAN_POINT('Ctrl Pts',(8.90000422571091,-1.53117752164703,0.692323975790708));
#10070=CARTESIAN_POINT('Ctrl Pts',(8.90000367147839,-1.52384911813356,0.695350638493274));
#10071=CARTESIAN_POINT('Ctrl Pts',(8.9000023358238,-1.51621796414731,0.697522741667433));
#10072=CARTESIAN_POINT('Ctrl Pts',(8.90000125519218,-1.50843132129101,0.698770821080692));
#10073=CARTESIAN_POINT('Ctrl Pts',(8.90000055451733,-1.5033825102871,0.699580068042664));
#10074=CARTESIAN_POINT('Ctrl Pts',(8.9,-1.49826772866746,0.7));
#10075=CARTESIAN_POINT('Ctrl Pts',(8.9,-1.49312521822106,0.7));
#10076=CARTESIAN_POINT('',(8.9,-1.62420669932031,0.));
#10077=CARTESIAN_POINT('Ctrl Pts',(8.9,-1.62420669932031,0.));
#10078=CARTESIAN_POINT('Ctrl Pts',(8.9,-1.61904139377919,0.100793652073202));
#10079=CARTESIAN_POINT('Ctrl Pts',(8.9,-1.61387638451174,0.201587891198165));
#10080=CARTESIAN_POINT('Ctrl Pts',(8.9,-1.60354122564866,0.403289532862703));
#10081=CARTESIAN_POINT('Ctrl Pts',(8.9,-1.59837101783099,0.50419808623799));
#10082=CARTESIAN_POINT('Ctrl Pts',(8.9,-1.59320117118329,0.605106081470792));
#10083=CARTESIAN_POINT('',(8.9,-1.68851851851852,0.));
#10084=CARTESIAN_POINT('Origin',(4.5,-1.48481481481482,0.));
#10085=CARTESIAN_POINT('',(4.5,1.41772989878425,0.));
#10086=CARTESIAN_POINT('',(4.5,-1.48481481481482,0.));
#10087=CARTESIAN_POINT('',(4.5,1.38566996325095,0.605286533624017));
#10088=CARTESIAN_POINT('Ctrl Pts',(4.5,1.38566996325095,0.605286533624017));
#10089=CARTESIAN_POINT('Ctrl Pts',(4.5,1.3910232158183,0.504222354021684));
#10090=CARTESIAN_POINT('Ctrl Pts',(4.5,1.39637635187357,0.403158168247774));
#10091=CARTESIAN_POINT('Ctrl Pts',(4.5,1.4070629957395,0.201395990303158));
#10092=CARTESIAN_POINT('Ctrl Pts',(4.5,1.41239650438775,0.100697998177668));
#10093=CARTESIAN_POINT('Ctrl Pts',(4.5,1.41772989878425,0.));
#10094=CARTESIAN_POINT('',(4.5,1.28575421950843,0.7));
#10095=CARTESIAN_POINT('Ctrl Pts',(4.5,1.28575421950843,0.7));
#10096=CARTESIAN_POINT('Ctrl Pts',(4.5,1.29366545802379,0.7));
#10097=CARTESIAN_POINT('Ctrl Pts',(4.50000067540813,1.30151306508378,0.699006020085879));
#10098=CARTESIAN_POINT('Ctrl Pts',(4.50000126278178,1.30915682219698,0.697118891599074));
#10099=CARTESIAN_POINT('Ctrl Pts',(4.50000159346398,1.31346013814185,0.696056467716811));
#10100=CARTESIAN_POINT('Ctrl Pts',(4.50000189442328,1.31769890045703,0.694709922559592));
#10101=CARTESIAN_POINT('Ctrl Pts',(4.50000208642664,1.32184639782974,0.693090275295953));
#10102=CARTESIAN_POINT('Ctrl Pts',(4.50000243009859,1.32927011415192,0.690191225399894));
#10103=CARTESIAN_POINT('Ctrl Pts',(4.50000235826664,1.33632110693134,0.686451804482762));
#10104=CARTESIAN_POINT('Ctrl Pts',(4.50000192249634,1.34285330390028,0.681953677325188));
#10105=CARTESIAN_POINT('Ctrl Pts',(4.5000016824508,1.3464515866709,0.679475868782656));
#10106=CARTESIAN_POINT('Ctrl Pts',(4.50000134086274,1.34989218134371,0.676766953538005));
#10107=CARTESIAN_POINT('Ctrl Pts',(4.50000103767597,1.35314674504257,0.67383503027087));
#10108=CARTESIAN_POINT('Ctrl Pts',(4.50000074242034,1.35631617169348,0.670979804009792));
#10109=CARTESIAN_POINT('Ctrl Pts',(4.50000047986374,1.35928994516467,0.667930335702103));
#10110=CARTESIAN_POINT('Ctrl Pts',(4.5000004798165,1.36204555935344,0.66469809744354));
#10111=CARTESIAN_POINT('Ctrl Pts',(4.5000004797289,1.36715559606013,0.658704204607119));
#10112=CARTESIAN_POINT('Ctrl Pts',(4.50000128456446,1.3715183542993,0.652083197653858));
#10113=CARTESIAN_POINT('Ctrl Pts',(4.50000155892095,1.37507421485048,0.645000595057188));
#10114=CARTESIAN_POINT('Ctrl Pts',(4.50000158702893,1.37543851484667,0.644274978272754));
#10115=CARTESIAN_POINT('Ctrl Pts',(4.50000161091379,1.37579430519483,0.643544496675346));
#10116=CARTESIAN_POINT('Ctrl Pts',(4.50000163009343,1.37614149316233,0.642809317076966));
#10117=CARTESIAN_POINT('Ctrl Pts',(4.50000181728783,1.37953006709248,0.635633923185928));
#10118=CARTESIAN_POINT('Ctrl Pts',(4.50000140772507,1.38206400387968,0.628095594687559));
#10119=CARTESIAN_POINT('Ctrl Pts',(4.50000081194859,1.38368993781387,0.620362729373495));
#10120=CARTESIAN_POINT('Ctrl Pts',(4.50000042990035,1.38473258588096,0.615403944208116));
#10121=CARTESIAN_POINT('Ctrl Pts',(4.49999999988018,1.38540098970406,0.610364492806037));
#10122=CARTESIAN_POINT('Ctrl Pts',(4.50000000014037,1.38566996330298,0.605286533623957));
#10123=CARTESIAN_POINT('',(4.5,-1.28575421950842,0.7));
#10124=CARTESIAN_POINT('',(4.5,-0.742407407407408,0.7));
#10125=CARTESIAN_POINT('',(4.5,-1.38566996325095,0.605286533624017));
#10126=CARTESIAN_POINT('Ctrl Pts',(4.50000000014037,-1.38566996330298,0.605286533623957));
#10127=CARTESIAN_POINT('Ctrl Pts',(4.49999999973491,-1.38525081272033,0.613199687771457));
#10128=CARTESIAN_POINT('Ctrl Pts',(4.50000095642016,-1.38386419754969,0.62102180968747));
#10129=CARTESIAN_POINT('Ctrl Pts',(4.50000138305812,-1.38159414679432,0.628592503408469));
#10130=CARTESIAN_POINT('Ctrl Pts',(4.50000162118259,-1.38032713666619,0.632818023740444));
#10131=CARTESIAN_POINT('Ctrl Pts',(4.50000172745986,-1.37878391728058,0.636965253716347));
#10132=CARTESIAN_POINT('Ctrl Pts',(4.50000166716583,-1.37697237493585,0.641004309729874));
#10133=CARTESIAN_POINT('Ctrl Pts',(4.50000155916287,-1.37372741146613,0.648239354085419));
#10134=CARTESIAN_POINT('Ctrl Pts',(4.50000084040372,-1.36965973349804,0.655049237033139));
#10135=CARTESIAN_POINT('Ctrl Pts',(4.50000056390271,-1.36483316768901,0.661270759279915));
#10136=CARTESIAN_POINT('Ctrl Pts',(4.50000051219424,-1.36393055121024,0.662434246679675));
#10137=CARTESIAN_POINT('Ctrl Pts',(4.50000048023544,-1.3630012658104,0.663577087492372));
#10138=CARTESIAN_POINT('Ctrl Pts',(4.50000048056391,-1.36204555937839,0.664698097443534));
#10139=CARTESIAN_POINT('Ctrl Pts',(4.50000048121673,-1.36014610273268,0.666926093123284));
#10140=CARTESIAN_POINT('Ctrl Pts',(4.50000060829837,-1.35814231322364,0.669067903674665));
#10141=CARTESIAN_POINT('Ctrl Pts',(4.50000078085101,-1.35604151212276,0.671119765431539));
#10142=CARTESIAN_POINT('Ctrl Pts',(4.50000124774248,-1.3503571825734,0.676671675324794));
#10143=CARTESIAN_POINT('Ctrl Pts',(4.50000197143062,-1.34402953514766,0.681505303070731));
#10144=CARTESIAN_POINT('Ctrl Pts',(4.50000220836427,-1.33722229030693,0.685566265232058));
#10145=CARTESIAN_POINT('Ctrl Pts',(4.50000235894787,-1.33289593407788,0.688147216755564));
#10146=CARTESIAN_POINT('Ctrl Pts',(4.50000234488938,-1.32837489877041,0.690415387400166));
#10147=CARTESIAN_POINT('Ctrl Pts',(4.50000216490635,-1.32369554581057,0.69234752884452));
#10148=CARTESIAN_POINT('Ctrl Pts',(4.50000188343739,-1.31637767466938,0.695369135087455));
#10149=CARTESIAN_POINT('Ctrl Pts',(4.50000119588393,-1.3087575932273,0.697536490026807));
#10150=CARTESIAN_POINT('Ctrl Pts',(4.50000064127173,-1.30098224657147,0.698779892333419));
#10151=CARTESIAN_POINT('Ctrl Pts',(4.50000028296845,-1.29595903898196,0.699583183579437));
#10152=CARTESIAN_POINT('Ctrl Pts',(4.5,-1.29087043558603,0.7));
#10153=CARTESIAN_POINT('Ctrl Pts',(4.5,-1.28575421950843,0.7));
#10154=CARTESIAN_POINT('',(4.5,-1.41772989878425,0.));
#10155=CARTESIAN_POINT('Ctrl Pts',(4.5,-1.41772989878425,0.));
#10156=CARTESIAN_POINT('Ctrl Pts',(4.5,-1.41239649634988,0.100698149937961));
#10157=CARTESIAN_POINT('Ctrl Pts',(4.5,-1.40706297966336,0.201396293824709));
#10158=CARTESIAN_POINT('Ctrl Pts',(4.5,-1.39637633579674,0.403158471769294));
#10159=CARTESIAN_POINT('Ctrl Pts',(4.5,-1.39102320777973,0.504222505781934));
#10160=CARTESIAN_POINT('Ctrl Pts',(4.5,-1.38566996325095,0.605286533624017));
#10161=CARTESIAN_POINT('',(4.5,-1.48481481481482,0.));
#10162=CARTESIAN_POINT('Origin',(1.1,-1.39290118819044,0.));
#10163=CARTESIAN_POINT('',(1.1,1.324891758307,0.));
#10164=CARTESIAN_POINT('',(1.1,-1.39290118819044,0.));
#10165=CARTESIAN_POINT('',(1.10000000295569,1.29254692766489,0.605334652628491));
#10166=CARTESIAN_POINT('Ctrl Pts',(1.10000000295569,1.29254692766489,0.605334652628491));
#10167=CARTESIAN_POINT('Ctrl Pts',(1.10000000295569,1.29794978210809,0.504228164786351));
#10168=CARTESIAN_POINT('Ctrl Pts',(1.1,1.30335245345465,0.403121008362245));
#10169=CARTESIAN_POINT('Ctrl Pts',(1.1,1.31413403739463,0.20134322693425));
#10170=CARTESIAN_POINT('Ctrl Pts',(1.1,1.31951302132877,0.100671299071668));
#10171=CARTESIAN_POINT('Ctrl Pts',(1.1,1.324891758307,0.));
#10172=CARTESIAN_POINT('Ctrl Pts',(1.1,1.19266190204553,0.7));
#10173=CARTESIAN_POINT('Ctrl Pts',(1.1,1.20057109129252,0.7));
#10174=CARTESIAN_POINT('Ctrl Pts',(1.10000046829629,1.20841685974333,0.699006220526237));
#10175=CARTESIAN_POINT('Ctrl Pts',(1.10000087277688,1.21605887983377,0.697119382842322));
#10176=CARTESIAN_POINT('Ctrl Pts',(1.10000109992184,1.22035042410288,0.696059787689036));
#10177=CARTESIAN_POINT('Ctrl Pts',(1.10000130563842,1.22457776983048,0.694717521940989));
#10178=CARTESIAN_POINT('Ctrl Pts',(1.10000143498593,1.22871439246446,0.693103507978966));
#10179=CARTESIAN_POINT('Ctrl Pts',(1.10000166711622,1.23613807995602,0.690206957744321));
#10180=CARTESIAN_POINT('Ctrl Pts',(1.10000160692769,1.24318920265812,0.686469797174223));
#10181=CARTESIAN_POINT('Ctrl Pts',(1.10000129432656,1.24972159507123,0.681973692132557));
#10182=CARTESIAN_POINT('Ctrl Pts',(1.10000112259081,1.25331033895651,0.679503636989594));
#10183=CARTESIAN_POINT('Ctrl Pts',(1.10000088087184,1.25674225826706,0.676803638555143));
#10184=CARTESIAN_POINT('Ctrl Pts',(1.10000066684112,1.25998923415267,0.673881729486736));
#10185=CARTESIAN_POINT('Ctrl Pts',(1.100000457217,1.26316935916797,0.671019978599686));
#10186=CARTESIAN_POINT('Ctrl Pts',(1.1000002715704,1.26615273734033,0.667962699881477));
#10187=CARTESIAN_POINT('Ctrl Pts',(1.1000002731257,1.2689166530284,0.664721467295484));
#10188=CARTESIAN_POINT('Ctrl Pts',(1.10000027600127,1.2740268283512,0.658728785663437));
#10189=CARTESIAN_POINT('Ctrl Pts',(1.10000085014601,1.27838972527875,0.652108677049879));
#10190=CARTESIAN_POINT('Ctrl Pts',(1.1000010530947,1.28194599975408,0.64502688444408));
#10191=CARTESIAN_POINT('Ctrl Pts',(1.10000107362034,1.2823056710724,0.644310652415237));
#10192=CARTESIAN_POINT('Ctrl Pts',(1.10000109127028,1.28265705236355,0.643589678557342));
#10193=CARTESIAN_POINT('Ctrl Pts',(1.10000110571348,1.28300005475086,0.642864123553892));
#10194=CARTESIAN_POINT('Ctrl Pts',(1.10000124853573,1.28639184812822,0.635689442715943));
#10195=CARTESIAN_POINT('Ctrl Pts',(1.10000097361067,1.28892914698194,0.628151301589031));
#10196=CARTESIAN_POINT('Ctrl Pts',(1.10000056283738,1.29055881622654,0.620418355899457));
#10197=CARTESIAN_POINT('Ctrl Pts',(1.10000029930222,1.29160434466024,0.615457217544876));
#10198=CARTESIAN_POINT('Ctrl Pts',(1.0999999999818,1.29227543558766,0.610415225971447));
#10199=CARTESIAN_POINT('Ctrl Pts',(1.1000000000255,1.29254692753179,0.605334652628598));
#10200=CARTESIAN_POINT('',(1.10000000295569,-1.29254692766489,0.605334652628491));
#10201=CARTESIAN_POINT('Ctrl Pts',(1.1000000000255,-1.29254692753179,0.605334652628598));
#10202=CARTESIAN_POINT('Ctrl Pts',(1.09999999995744,-1.29212405100831,0.613248166229861));
#10203=CARTESIAN_POINT('Ctrl Pts',(1.10000066442022,-1.29073420569755,0.621070584654331));
#10204=CARTESIAN_POINT('Ctrl Pts',(1.10000095378343,-1.28846118610397,0.628641296001913));
#10205=CARTESIAN_POINT('Ctrl Pts',(1.10000111506646,-1.28719426797524,0.632861000698125));
#10206=CARTESIAN_POINT('Ctrl Pts',(1.10000118318417,-1.28565198202118,0.637002542581089));
#10207=CARTESIAN_POINT('Ctrl Pts',(1.10000113489265,-1.28384214455607,0.641036116698538));
#10208=CARTESIAN_POINT('Ctrl Pts',(1.10000104828677,-1.28059638744501,0.648269916488365));
#10209=CARTESIAN_POINT('Ctrl Pts',(1.10000053334783,-1.27652829029495,0.655078571385522));
#10210=CARTESIAN_POINT('Ctrl Pts',(1.10000033433257,-1.27170133822839,0.661298646557671));
#10211=CARTESIAN_POINT('Ctrl Pts',(1.10000029715544,-1.27079963749419,0.662460590217389));
#10212=CARTESIAN_POINT('Ctrl Pts',(1.10000027400485,-1.26987132743055,0.663601924550879));
#10213=CARTESIAN_POINT('Ctrl Pts',(1.10000027368829,-1.26891665304159,0.664721467295481));
#10214=CARTESIAN_POINT('Ctrl Pts',(1.10000027305905,-1.2670190620795,0.666946764442229));
#10215=CARTESIAN_POINT('Ctrl Pts',(1.10000036187052,-1.26501734165944,0.669086014589825));
#10216=CARTESIAN_POINT('Ctrl Pts',(1.10000048327469,-1.26291879257262,0.671135465892351));
#10217=CARTESIAN_POINT('Ctrl Pts',(1.10000081209565,-1.25723491092676,0.676686367091516));
#10218=CARTESIAN_POINT('Ctrl Pts',(1.10000132622062,-1.25090760500066,0.68151881845922));
#10219=CARTESIAN_POINT('Ctrl Pts',(1.10000150097561,-1.24410063152763,0.68557843671136));
#10220=CARTESIAN_POINT('Ctrl Pts',(1.10000161196703,-1.2397773464179,0.688156805381407));
#10221=CARTESIAN_POINT('Ctrl Pts',(1.1000016084534,-1.23525961544019,0.690422742497405));
#10222=CARTESIAN_POINT('Ctrl Pts',(1.10000148831111,-1.23058375131837,0.692353039195786));
#10223=CARTESIAN_POINT('Ctrl Pts',(1.10000130031927,-1.22326722442338,0.695373457954986));
#10224=CARTESIAN_POINT('Ctrl Pts',(1.1000008264887,-1.21564857658641,0.697539632783775));
#10225=CARTESIAN_POINT('Ctrl Pts',(1.10000044322439,-1.20787483729518,0.698781928831272));
#10226=CARTESIAN_POINT('Ctrl Pts',(1.1000001958084,-1.20285650563037,0.6995838921283));
#10227=CARTESIAN_POINT('Ctrl Pts',(1.1,-1.19777295102175,0.7));
#10228=CARTESIAN_POINT('Ctrl Pts',(1.1,-1.19266190204553,0.7));
#10229=CARTESIAN_POINT('',(1.1,-1.324891758307,0.));
#10230=CARTESIAN_POINT('Ctrl Pts',(1.1,-1.324891758307,0.));
#10231=CARTESIAN_POINT('Ctrl Pts',(1.1,-1.3195129727271,0.10067220872632));
#10232=CARTESIAN_POINT('Ctrl Pts',(1.1,-1.31413394019217,0.201345046154956));
#10233=CARTESIAN_POINT('Ctrl Pts',(1.1,-1.30335235623932,0.40312282767794));
#10234=CARTESIAN_POINT('Ctrl Pts',(1.10000000295569,-1.29794973349953,0.504229074424201));
#10235=CARTESIAN_POINT('Ctrl Pts',(1.10000000295569,-1.29254692766489,0.605334652628491));
#10236=CARTESIAN_POINT('',(1.1,-1.39290118819044,0.));
#10237=CARTESIAN_POINT('Origin',(0.199725906950915,-1.5,-0.0104671912485888));
#10238=CARTESIAN_POINT('',(0.200274469199584,1.20659878095028,0.));
#10239=CARTESIAN_POINT('',(0.200274469199585,-0.75,0.));
#10240=CARTESIAN_POINT('',(0.231993417893744,1.17491202960101,0.605233595624295));
#10241=CARTESIAN_POINT('Ctrl Pts',(0.200274469199584,1.20659878095028,-9.43255890062389E-18));
#10242=CARTESIAN_POINT('Ctrl Pts',(0.210847451958254,1.19603647956141,0.20174452921517));
#10243=CARTESIAN_POINT('Ctrl Pts',(0.221420434855641,1.18547422886796,0.403489061077219));
#10244=CARTESIAN_POINT('Ctrl Pts',(0.231993417893744,1.17491202960101,0.605233595624295));
#10245=CARTESIAN_POINT('',(0.231993417893744,-1.17491202960101,0.605233595624295));
#10246=CARTESIAN_POINT('',(0.231993417893744,-0.75,0.605233595624295));
#10247=CARTESIAN_POINT('',(0.200274469199584,-1.20659878095028,1.38777878078145E-17));
#10248=CARTESIAN_POINT('Ctrl Pts',(0.231993417893744,-1.17491202960101,
0.605233595624295));
#10249=CARTESIAN_POINT('Ctrl Pts',(0.221420434855641,-1.18547422886796,
0.40348906107722));
#10250=CARTESIAN_POINT('Ctrl Pts',(0.210847451958254,-1.19603647956141,
0.20174452921517));
#10251=CARTESIAN_POINT('Ctrl Pts',(0.200274469199584,-1.20659878095028,
2.0491421059976E-17));
#10252=CARTESIAN_POINT('',(0.200274469199585,-0.75,0.));
#10253=CARTESIAN_POINT('Origin',(6.87299528185878,-3.57834294608796E-18,
0.));
#10254=CARTESIAN_POINT('Ctrl Pts',(8.90000000000001,-1.62420669932031,-3.75133951679985E-17));
#10255=CARTESIAN_POINT('Ctrl Pts',(10.0682843079684,-1.69891080436391,-1.31961514553165E-7));
#10256=CARTESIAN_POINT('Ctrl Pts',(11.2345361392062,-1.79243531443695,-6.44452192334729E-8));
#10257=CARTESIAN_POINT('Ctrl Pts',(12.4000000002382,-1.91212902541327,2.95121624705651E-11));
#10258=CARTESIAN_POINT('Ctrl Pts',(12.4000000002382,1.91212902541327,2.95118849063386E-11));
#10259=CARTESIAN_POINT('Ctrl Pts',(11.2345361911441,1.79243531977099,-6.4445136166539E-8));
#10260=CARTESIAN_POINT('Ctrl Pts',(10.0682843567552,1.69891080748336,-1.31958638870612E-7));
#10261=CARTESIAN_POINT('Ctrl Pts',(8.9,1.62420669932031,6.39679281766448E-17));
#10262=CARTESIAN_POINT('',(8.7,1.61160179736194,0.));
#10263=CARTESIAN_POINT('',(8.7,1.68851851851852,0.));
#10264=CARTESIAN_POINT('Ctrl Pts',(8.70000000002062,1.61160179731554,-3.21507306454832E-13));
#10265=CARTESIAN_POINT('Ctrl Pts',(7.99734938728961,1.56795839277283,5.29471456843263E-9));
#10266=CARTESIAN_POINT('Ctrl Pts',(7.29393815910572,1.53097060499506,-6.44604909847991E-9));
#10267=CARTESIAN_POINT('Ctrl Pts',(6.58949465297818,1.49904250536939,-7.60372244394637E-9));
#10268=CARTESIAN_POINT('Ctrl Pts',(5.94302350041144,1.46974193664425,-8.66612477447903E-9));
#10269=CARTESIAN_POINT('Ctrl Pts',(5.29757001768168,1.44478244743454,1.79883147367388E-8));
#10270=CARTESIAN_POINT('Ctrl Pts',(4.65216233480351,1.42284617839366,3.84107779578714E-9));
#10271=CARTESIAN_POINT('Ctrl Pts',(4.60144142975536,1.4211222642714,2.72928337404163E-9));
#10272=CARTESIAN_POINT('Ctrl Pts',(4.55072080855761,1.41941704699729,1.44770501019496E-9));
#10273=CARTESIAN_POINT('Ctrl Pts',(4.50000000001737,1.41772989873549,-1.00876616052154E-12));
#10274=CARTESIAN_POINT('',(4.3,1.41116952203211,0.));
#10275=CARTESIAN_POINT('',(4.3,1.48481481481482,0.));
#10276=CARTESIAN_POINT('Ctrl Pts',(4.3,1.41116952203211,-1.0790522121662E-15));
#10277=CARTESIAN_POINT('Ctrl Pts',(3.23514221724601,1.37672428690534,3.20725535317031E-8));
#10278=CARTESIAN_POINT('Ctrl Pts',(2.16992716239601,1.34987955958158,4.63097810372671E-9));
#10279=CARTESIAN_POINT('Ctrl Pts',(1.10000000020726,1.32489175811528,-9.82792569252214E-12));
#10280=CARTESIAN_POINT('',(0.9,1.32024227787037,0.));
#10281=CARTESIAN_POINT('',(0.9,1.39290118819044,0.));
#10282=CARTESIAN_POINT('',(0.297857995688647,1.306435779838,0.));
#10283=CARTESIAN_POINT('Ctrl Pts',(0.9,1.32024227787037,-6.93889390390723E-18));
#10284=CARTESIAN_POINT('Ctrl Pts',(0.699470323836888,1.31560060380002,-4.72996299588896E-10));
#10285=CARTESIAN_POINT('Ctrl Pts',(0.498765843889866,1.3110112408976,-1.02277582142263E-13));
#10286=CARTESIAN_POINT('Ctrl Pts',(0.297857995688647,1.306435779838,-1.00157829096748E-16));
#10287=CARTESIAN_POINT('Ctrl Pts',(0.297857995688647,1.306435779838,-1.95156391047391E-17));
#10288=CARTESIAN_POINT('Ctrl Pts',(0.289922476296638,1.30625505685688,-1.46278605970555E-13));
#10289=CARTESIAN_POINT('Ctrl Pts',(0.282050301799808,1.30510306275878,-1.25203502999379E-6));
#10290=CARTESIAN_POINT('Ctrl Pts',(0.274405144964298,1.30305953674341,-1.39678564665046E-6));
#10291=CARTESIAN_POINT('Ctrl Pts',(0.269498922713003,1.30174811919849,-1.48967827287246E-6));
#10292=CARTESIAN_POINT('Ctrl Pts',(0.26468600784495,1.30006837070384,-1.17796618578504E-6));
#10293=CARTESIAN_POINT('Ctrl Pts',(0.260012701218123,1.29803054880949,-5.63923085528507E-7));
#10294=CARTESIAN_POINT('Ctrl Pts',(0.252740988282594,1.29485967708789,3.91534262267771E-7));
#10295=CARTESIAN_POINT('Ctrl Pts',(0.245891302634708,1.2908611961912,2.26944434681222E-6));
#10296=CARTESIAN_POINT('Ctrl Pts',(0.239629152465829,1.28609427281,1.73040332626933E-6));
#10297=CARTESIAN_POINT('Ctrl Pts',(0.238677421334952,1.28536978852616,1.6484790500646E-6));
#10298=CARTESIAN_POINT('Ctrl Pts',(0.23773930716971,1.28462746803483,1.50379952206709E-6));
#10299=CARTESIAN_POINT('Ctrl Pts',(0.236815449960777,1.28386742955246,1.27686598471174E-6));
#10300=CARTESIAN_POINT('Ctrl Pts',(0.233849259515119,1.28142720517261,5.48259784756267E-7));
#10301=CARTESIAN_POINT('Ctrl Pts',(0.231029859162728,1.27880446664625,-1.01231737317126E-6));
#10302=CARTESIAN_POINT('Ctrl Pts',(0.228365947504865,1.27601569667724,-2.73789903475208E-6));
#10303=CARTESIAN_POINT('Ctrl Pts',(0.222875659368053,1.2702680771449,-6.2943009513513E-6));
#10304=CARTESIAN_POINT('Ctrl Pts',(0.218108003769119,1.26388547870891,-1.02458913084139E-5));
#10305=CARTESIAN_POINT('Ctrl Pts',(0.214119068651703,1.25703104885628,-1.16727273233865E-5));
#10306=CARTESIAN_POINT('Ctrl Pts',(0.211608035823831,1.25271618840614,-1.25709199407453E-5));
#10307=CARTESIAN_POINT('Ctrl Pts',(0.209406266788438,1.24821342134138,-1.25531979180244E-5));
#10308=CARTESIAN_POINT('Ctrl Pts',(0.207536767894457,1.24355803714115,-1.16467700682383E-5));
#10309=CARTESIAN_POINT('Ctrl Pts',(0.204585779527196,1.23620955211972,-1.02159812889057E-5));
#10310=CARTESIAN_POINT('Ctrl Pts',(0.20249437279756,1.22856635796309,-6.44823334219156E-6));
#10311=CARTESIAN_POINT('Ctrl Pts',(0.201333199355162,1.22077498745768,-3.37414558979738E-6));
#10312=CARTESIAN_POINT('Ctrl Pts',(0.200635497716839,1.21609347152911,-1.5270519663277E-6));
#10313=CARTESIAN_POINT('Ctrl Pts',(0.200274469246579,1.21135795995708,-3.76748562593766E-12));
#10314=CARTESIAN_POINT('Ctrl Pts',(0.200274469199584,1.20659878095028,6.07153216591882E-18));
#10315=CARTESIAN_POINT('',(-2.81723893694256E-19,1.20714678905882,-2.77862675945125E-17));
#10316=CARTESIAN_POINT('',(0.,-1.5,0.));
#10317=CARTESIAN_POINT('',(0.292751161823634,1.50665779898694,0.));
#10318=CARTESIAN_POINT('Ctrl Pts',(0.292751161823634,1.50665779898694,-4.77048955893622E-17));
#10319=CARTESIAN_POINT('Ctrl Pts',(0.274916014309114,1.50625165707847,3.84528327419955E-12));
#10320=CARTESIAN_POINT('Ctrl Pts',(0.257184594685611,1.50420857033458,-2.03607170333744E-6));
#10321=CARTESIAN_POINT('Ctrl Pts',(0.239764500086274,1.50063675387888,-2.79213621391921E-6));
#10322=CARTESIAN_POINT('Ctrl Pts',(0.222116086584643,1.49701812291205,-3.55811018958082E-6));
#10323=CARTESIAN_POINT('Ctrl Pts',(0.204785660682177,1.49183000356027,-2.9511242418033E-6));
#10324=CARTESIAN_POINT('Ctrl Pts',(0.187998620502071,1.4851341555102,-6.80337370794577E-7));
#10325=CARTESIAN_POINT('Ctrl Pts',(0.185044527596802,1.48395585623842,-2.80736529130144E-7));
#10326=CARTESIAN_POINT('Ctrl Pts',(0.182107319868513,1.48273075079643,1.61255976403501E-7));
#10327=CARTESIAN_POINT('Ctrl Pts',(0.17918831289364,1.48145903083089,6.35063889779883E-7));
#10328=CARTESIAN_POINT('Ctrl Pts',(0.162608037952008,1.47423552404966,3.32634402063389E-6));
#10329=CARTESIAN_POINT('Ctrl Pts',(0.146760254055949,1.46557586252388,7.36741945499403E-6));
#10330=CARTESIAN_POINT('Ctrl Pts',(0.131860714325404,1.4555643673366,8.80872142158042E-6));
#10331=CARTESIAN_POINT('Ctrl Pts',(0.12416804976458,1.45039541073654,9.55286874158632E-6));
#10332=CARTESIAN_POINT('Ctrl Pts',(0.116728404005452,1.44486529627202,9.54902993357918E-6));
#10333=CARTESIAN_POINT('Ctrl Pts',(0.109574210210226,1.43898090192647,7.86258910610491E-6));
#10334=CARTESIAN_POINT('Ctrl Pts',(0.100675189791982,1.43166137062374,5.76484451217541E-6));
#10335=CARTESIAN_POINT('Ctrl Pts',(0.0922175942578585,1.42379373777092,
1.07962821494929E-6));
#10336=CARTESIAN_POINT('Ctrl Pts',(0.0842272493232774,1.41542759110015,
-4.17082519724513E-6));
#10337=CARTESIAN_POINT('Ctrl Pts',(0.0719003514327883,1.40252093480537,
-1.22708263387205E-5));
#10338=CARTESIAN_POINT('Ctrl Pts',(0.0607923942774574,1.38854365509349,
-2.1446290640466E-5));
#10339=CARTESIAN_POINT('Ctrl Pts',(0.0509667079859164,1.37370740939602,
-2.73088451608079E-5));
#10340=CARTESIAN_POINT('Ctrl Pts',(0.040988527714452,1.35864090617899,-3.32623861267576E-5));
#10341=CARTESIAN_POINT('Ctrl Pts',(0.0323319291028794,1.34268723517955,
-3.58272570146011E-5));
#10342=CARTESIAN_POINT('Ctrl Pts',(0.0251054147216294,1.32603775378173,
-3.42048160832586E-5));
#10343=CARTESIAN_POINT('Ctrl Pts',(0.0239557673766072,1.32338903116455,
-3.39467061825833E-5));
#10344=CARTESIAN_POINT('Ctrl Pts',(0.022842414085455,1.32072266145131,-3.35898145907185E-5));
#10345=CARTESIAN_POINT('Ctrl Pts',(0.0217659098422027,1.31803938112476,
-3.31388957009043E-5));
#10346=CARTESIAN_POINT('Ctrl Pts',(0.0146851456525434,1.30038996137917,
-3.01729526055095E-5));
#10347=CARTESIAN_POINT('Ctrl Pts',(0.00925910545076598,1.282173175788,-2.28911926108039E-5));
#10348=CARTESIAN_POINT('Ctrl Pts',(0.0055880418397064,1.26361786690427,
-1.53360241296986E-5));
#10349=CARTESIAN_POINT('Ctrl Pts',(0.00217213684284492,1.24635225152695,
-8.30598038733772E-6));
#10350=CARTESIAN_POINT('Ctrl Pts',(0.000275638047107462,1.2287919996398,
-1.11502351997496E-6));
#10351=CARTESIAN_POINT('Ctrl Pts',(2.78020181985954E-5,1.21111091902543,
-1.13803743790751E-7));
#10352=CARTESIAN_POINT('Ctrl Pts',(9.289355304618E-6,1.20979019141994,-3.90154078055202E-8));
#10353=CARTESIAN_POINT('Ctrl Pts',(3.5054796412911E-11,1.20846879032832,
-2.82152417201308E-12));
#10354=CARTESIAN_POINT('Ctrl Pts',(6.5594231435373E-18,1.20714678905882,
2.42861286636753E-17));
#10355=CARTESIAN_POINT('',(12.8678148030684,2.16300527278356,0.));
#10356=CARTESIAN_POINT('Ctrl Pts',(0.292751161823634,1.50665779898694,0.));
#10357=CARTESIAN_POINT('Ctrl Pts',(4.48443904223854,1.60211086545473,0.));
#10358=CARTESIAN_POINT('Ctrl Pts',(8.67612692265345,1.70561506876628,0.));
#10359=CARTESIAN_POINT('Ctrl Pts',(12.8678148030684,2.16300527278356,0.));
#10360=CARTESIAN_POINT('',(13.2,1.86519007666192,1.29914761427265E-16));
#10361=CARTESIAN_POINT('Ctrl Pts',(13.2,1.86519007666192,1.40512601554121E-16));
#10362=CARTESIAN_POINT('Ctrl Pts',(13.2000000013352,1.88296731840607,9.35191444695304E-11));
#10363=CARTESIAN_POINT('Ctrl Pts',(13.1983511006715,1.90064589040826,-4.81925060583158E-6));
#10364=CARTESIAN_POINT('Ctrl Pts',(13.1951709302004,1.91804121845656,-9.22684518112407E-6));
#10365=CARTESIAN_POINT('Ctrl Pts',(13.1919252271695,1.93579500539423,-1.37252653764835E-5));
#10366=CARTESIAN_POINT('Ctrl Pts',(13.1870840836913,1.95325521073227,-1.77396479500911E-5));
#10367=CARTESIAN_POINT('Ctrl Pts',(13.1807207319279,1.9702167899609,-1.88895599539727E-5));
#10368=CARTESIAN_POINT('Ctrl Pts',(13.179605107926,1.97319049715201,-1.90911627380646E-5));
#10369=CARTESIAN_POINT('Ctrl Pts',(13.1784425783122,1.97614882406338,-1.92137058190342E-5));
#10370=CARTESIAN_POINT('Ctrl Pts',(13.1772333926356,1.97909058504493,-1.92562174744009E-5));
#10371=CARTESIAN_POINT('Ctrl Pts',(13.1703491364924,1.99583891121373,-1.94982490583826E-5));
#10372=CARTESIAN_POINT('Ctrl Pts',(13.1620175712498,2.0119031422279,-1.67925698753361E-5));
#10373=CARTESIAN_POINT('Ctrl Pts',(13.1523342210936,2.02708796667103,-1.30402710852334E-5));
#10374=CARTESIAN_POINT('Ctrl Pts',(13.1443502942575,2.03960786168842,-9.94649893779315E-6));
#10375=CARTESIAN_POINT('Ctrl Pts',(13.1354462980072,2.05153020544825,-6.18593217696112E-6));
#10376=CARTESIAN_POINT('Ctrl Pts',(13.1256528604983,2.06273196126272,-4.73977425690188E-6));
#10377=CARTESIAN_POINT('Ctrl Pts',(13.1217453950533,2.06720132901318,-4.16277439392992E-6));
#10378=CARTESIAN_POINT('Ctrl Pts',(13.1176961215346,2.07155579183536,-3.97575052791371E-6));
#10379=CARTESIAN_POINT('Ctrl Pts',(13.1135113749213,2.07579033931164,-3.99023031318383E-6));
#10380=CARTESIAN_POINT('Ctrl Pts',(13.1009362730034,2.08851509208914,-4.03374185458576E-6));
#10381=CARTESIAN_POINT('Ctrl Pts',(13.0872516297578,2.10004749226926,-5.60236028337187E-6));
#10382=CARTESIAN_POINT('Ctrl Pts',(13.0726646436523,2.11028882659185,-6.03124820804926E-6));
#10383=CARTESIAN_POINT('Ctrl Pts',(13.0580194031224,2.12057106059247,-6.46184893473862E-6));
#10384=CARTESIAN_POINT('Ctrl Pts',(13.0424632957183,2.12955278528135,-5.76500392338198E-6));
#10385=CARTESIAN_POINT('Ctrl Pts',(13.0261754841647,2.13709349482706,-4.98347139369932E-6));
#10386=CARTESIAN_POINT('Ctrl Pts',(13.0233759049672,2.13838960594114,-4.84914013593099E-6));
#10387=CARTESIAN_POINT('Ctrl Pts',(13.0205546633935,2.13964302898522,-4.72077764982159E-6));
#10388=CARTESIAN_POINT('Ctrl Pts',(13.0177126224567,2.14085289970554,-4.61407510358037E-6));
#10389=CARTESIAN_POINT('Ctrl Pts',(13.0148367726024,2.14207716304734,-4.50610322390289E-6));
#10390=CARTESIAN_POINT('Ctrl Pts',(13.0119432782921,2.14325527660784,-4.42172619954107E-6));
#10391=CARTESIAN_POINT('Ctrl Pts',(13.0090331608036,2.14438664763146,-4.38057543634576E-6));
#10392=CARTESIAN_POINT('Ctrl Pts',(12.9922536897216,2.1509100294015,-4.14330390220891E-6));
#10393=CARTESIAN_POINT('Ctrl Pts',(12.9749229882599,2.15588345271621,-5.05640020348117E-6));
#10394=CARTESIAN_POINT('Ctrl Pts',(12.9572550825995,2.15928949382789,-4.85686529648217E-6));
#10395=CARTESIAN_POINT('Ctrl Pts',(12.9529252316797,2.16012420794307,-4.80796553341985E-6));
#10396=CARTESIAN_POINT('Ctrl Pts',(12.9485750628159,2.16086455090717,-4.70814629363608E-6));
#10397=CARTESIAN_POINT('Ctrl Pts',(12.944207640703,2.16150979950679,-4.55317442353944E-6));
#10398=CARTESIAN_POINT('Ctrl Pts',(12.9263774359968,2.16414405704371,-3.92049452767182E-6));
#10399=CARTESIAN_POINT('Ctrl Pts',(12.9083632163621,2.16518216214944,-2.15504024707585E-6));
#10400=CARTESIAN_POINT('Ctrl Pts',(12.8903762705535,2.16459816844574,-9.12104093693782E-7));
#10401=CARTESIAN_POINT('Ctrl Pts',(12.8828459063217,2.16435367528137,-3.91739933400607E-7));
#10402=CARTESIAN_POINT('Ctrl Pts',(12.8753202361859,2.1638242536466,5.87463683432524E-12));
#10403=CARTESIAN_POINT('Ctrl Pts',(12.8678148030684,2.16300527278357,2.8796409701215E-16));
#10404=CARTESIAN_POINT('',(13.2,-1.86519007666192,1.11326398357188E-16));
#10405=CARTESIAN_POINT('',(13.2,2.2,0.));
#10406=CARTESIAN_POINT('',(12.8678148030684,-2.16300527278356,1.38777878078145E-17));
#10407=CARTESIAN_POINT('Ctrl Pts',(12.8678148030684,-2.16300527278357,2.56739074444567E-16));
#10408=CARTESIAN_POINT('Ctrl Pts',(12.8854929372559,-2.16493428409685,8.24591542686399E-11));
#10409=CARTESIAN_POINT('Ctrl Pts',(12.9032520674897,-2.16521372082443,-4.52295339524789E-6));
#10410=CARTESIAN_POINT('Ctrl Pts',(12.9208958607904,-2.1639404182545,-8.68231213275745E-6));
#10411=CARTESIAN_POINT('Ctrl Pts',(12.9389012534027,-2.16264102008682,-1.29269145154966E-5));
#10412=CARTESIAN_POINT('Ctrl Pts',(12.9567880250381,-2.15972433317902,-1.67278855193166E-5));
#10413=CARTESIAN_POINT('Ctrl Pts',(12.9743443410528,-2.15524079327399,-1.78237954457702E-5));
#10414=CARTESIAN_POINT('Ctrl Pts',(12.9774431846623,-2.15444940919484,-1.80172331504298E-5));
#10415=CARTESIAN_POINT('Ctrl Pts',(12.9805316913262,-2.15360908525727,-1.81351031595367E-5));
#10416=CARTESIAN_POINT('Ctrl Pts',(12.9836086301392,-2.15271994254544,-1.81766625580856E-5));
#10417=CARTESIAN_POINT('Ctrl Pts',(13.0010041030966,-2.14769317440371,-1.84116186093898E-5));
#10418=CARTESIAN_POINT('Ctrl Pts',(13.017876958431,-2.14115457229109,-1.5854618169158E-5));
#10419=CARTESIAN_POINT('Ctrl Pts',(13.0340226638693,-2.13317744288338,-1.23136839993165E-5));
#10420=CARTESIAN_POINT('Ctrl Pts',(13.0473215411186,-2.12660684953271,-9.39709115965876E-6));
#10421=CARTESIAN_POINT('Ctrl Pts',(13.060127470267,-2.11905920305061,-5.85016632862467E-6));
#10422=CARTESIAN_POINT('Ctrl Pts',(13.0723151314263,-2.11055132433008,-4.53327195050794E-6));
#10423=CARTESIAN_POINT('Ctrl Pts',(13.0772147086919,-2.10713106111368,-4.00386555564548E-6));
#10424=CARTESIAN_POINT('Ctrl Pts',(13.0820141951123,-2.10355537352593,-3.85636210984559E-6));
#10425=CARTESIAN_POINT('Ctrl Pts',(13.0867078006727,-2.0998301147952,-3.90248451975241E-6));
#10426=CARTESIAN_POINT('Ctrl Pts',(13.1007249787291,-2.08870484782034,-4.04022639510273E-6));
#10427=CARTESIAN_POINT('Ctrl Pts',(13.1136765748478,-2.07634683247102,-5.5945154994439E-6));
#10428=CARTESIAN_POINT('Ctrl Pts',(13.1254414850725,-2.06295113861397,-5.97495381195624E-6));
#10429=CARTESIAN_POINT('Ctrl Pts',(13.1372476314214,-2.04950849272046,-6.35672556443159E-6));
#10430=CARTESIAN_POINT('Ctrl Pts',(13.1478597809499,-2.03501968083851,-5.56609061204695E-6));
#10431=CARTESIAN_POINT('Ctrl Pts',(13.1571184147632,-2.01964723728874,-4.75455255839871E-6));
#10432=CARTESIAN_POINT('Ctrl Pts',(13.158708901902,-2.01700649414547,-4.61514313115074E-6));
#10433=CARTESIAN_POINT('Ctrl Pts',(13.1602593369672,-2.01433961799121,-4.48389992381974E-6));
#10434=CARTESIAN_POINT('Ctrl Pts',(13.1617687665475,-2.01164737048868,-4.37752847101542E-6));
#10435=CARTESIAN_POINT('Ctrl Pts',(13.1632768494098,-2.00895752501823,-4.27125192317111E-6));
#10436=CARTESIAN_POINT('Ctrl Pts',(13.164742106841,-2.00624572954308,-4.19089851494128E-6));
#10437=CARTESIAN_POINT('Ctrl Pts',(13.1661638648313,-2.00351289682408,-4.15637526360595E-6));
#10438=CARTESIAN_POINT('Ctrl Pts',(13.1744716670281,-1.98754405133797,-3.95464448717833E-6));
#10439=CARTESIAN_POINT('Ctrl Pts',(13.181298057795,-1.97085874357403,-5.01850453361653E-6));
#10440=CARTESIAN_POINT('Ctrl Pts',(13.1866022393826,-1.95366776591112,-4.89891140766866E-6));
#10441=CARTESIAN_POINT('Ctrl Pts',(13.1879075264936,-1.94943729958961,-4.86948116225E-6));
#10442=CARTESIAN_POINT('Ctrl Pts',(13.1891204013114,-1.94517611908519,-4.78523710928743E-6));
#10443=CARTESIAN_POINT('Ctrl Pts',(13.1902397948733,-1.94088722910442,-4.64104147683466E-6));
#10444=CARTESIAN_POINT('Ctrl Pts',(13.1947901580114,-1.92345278286841,-4.05488258426869E-6));
#10445=CARTESIAN_POINT('Ctrl Pts',(13.1977733658442,-1.90566244769967,-2.24449026644408E-6));
#10446=CARTESIAN_POINT('Ctrl Pts',(13.1991406030032,-1.88772335428786,-9.50757284845071E-7));
#10447=CARTESIAN_POINT('Ctrl Pts',(13.1997114533543,-1.8802334044254,-4.10596478211383E-7));
#10448=CARTESIAN_POINT('Ctrl Pts',(13.2000000000958,-1.87271737110067,6.9401096738129E-12));
#10449=CARTESIAN_POINT('Ctrl Pts',(13.2,-1.86519007666192,1.81278603239576E-16));
#10450=CARTESIAN_POINT('',(0.292751161823634,-1.50665779898694,-1.38777878078145E-17));
#10451=CARTESIAN_POINT('Ctrl Pts',(12.8678148030684,-2.16300527278356,0.));
#10452=CARTESIAN_POINT('Ctrl Pts',(8.67612692265345,-1.70561506876628,0.));
#10453=CARTESIAN_POINT('Ctrl Pts',(4.48443904223854,-1.60211086545473,0.));
#10454=CARTESIAN_POINT('Ctrl Pts',(0.292751161823634,-1.50665779898694,
0.));
#10455=CARTESIAN_POINT('',(4.02814324098787E-18,-1.20714678905882,5.54818711994559E-17));
#10456=CARTESIAN_POINT('Ctrl Pts',(-2.22044604925031E-16,-1.20714678905882,
-3.98986399474666E-17));
#10457=CARTESIAN_POINT('Ctrl Pts',(2.12382277713531E-10,-1.2249878157372,
-1.35440422383976E-12));
#10458=CARTESIAN_POINT('Ctrl Pts',(0.00163882612763064,-1.24276245549475,
-1.96699749426327E-6));
#10459=CARTESIAN_POINT('Ctrl Pts',(0.00481304415265273,-1.26026068126938,
-2.66007142975038E-6));
#10460=CARTESIAN_POINT('Ctrl Pts',(0.00802873944670128,-1.27798755504872,
-3.36220171040687E-6));
#10461=CARTESIAN_POINT('Ctrl Pts',(0.0128206026099745,-1.29543230475431,
-2.69550948014298E-6));
#10462=CARTESIAN_POINT('Ctrl Pts',(0.0191320595672371,-1.31236817798419,
-4.00401478067381E-7));
#10463=CARTESIAN_POINT('Ctrl Pts',(0.0202443702650641,-1.31535290133701,
4.0809101773195E-9));
#10464=CARTESIAN_POINT('Ctrl Pts',(0.0214039964883031,-1.3183217636574,
4.5005107558061E-7));
#10465=CARTESIAN_POINT('Ctrl Pts',(0.0226107760969305,-1.32127343934773,
9.26779280916758E-7));
#10466=CARTESIAN_POINT('Ctrl Pts',(0.0294548697216842,-1.33801348419941,
3.63048130534217E-6));
#10467=CARTESIAN_POINT('Ctrl Pts',(0.0377511831708778,-1.35405403406083,
7.64722139837078E-6));
#10468=CARTESIAN_POINT('Ctrl Pts',(0.0474204318104353,-1.36917746582299,
9.03443059383348E-6));
#10469=CARTESIAN_POINT('Ctrl Pts',(0.0524109755304394,-1.37698305136733,
9.75040433665629E-6));
#10470=CARTESIAN_POINT('Ctrl Pts',(0.0577680562174045,-1.38454410063597,
9.71159147480002E-6));
#10471=CARTESIAN_POINT('Ctrl Pts',(0.0634855547170043,-1.39182806229354,
7.98761394269614E-6));
#10472=CARTESIAN_POINT('Ctrl Pts',(0.0706048733905122,-1.40089791062835,
5.84095042579577E-6));
#10473=CARTESIAN_POINT('Ctrl Pts',(0.0782829434694699,-1.40953838460506,
1.09773645972912E-6));
#10474=CARTESIAN_POINT('Ctrl Pts',(0.0864706998703675,-1.41772246232928,
-4.21049985396393E-6));
#10475=CARTESIAN_POINT('Ctrl Pts',(0.0990944981487371,-1.43034058886193,
-1.2394683793612E-5));
#10476=CARTESIAN_POINT('Ctrl Pts',(0.112816484288725,-1.44176429483685,
-2.16481703631134E-5));
#10477=CARTESIAN_POINT('Ctrl Pts',(0.127426518150943,-1.45192534842919,
-2.7562374581111E-5));
#10478=CARTESIAN_POINT('Ctrl Pts',(0.142261949549145,-1.46224316253723,
-3.35678206860622E-5));
#10479=CARTESIAN_POINT('Ctrl Pts',(0.158014355623482,-1.47125989363127,
-3.6155642403295E-5));
#10480=CARTESIAN_POINT('Ctrl Pts',(0.17449494651519,-1.47886261331763,-3.45187637154371E-5));
#10481=CARTESIAN_POINT('Ctrl Pts',(0.177115379630184,-1.48007145458801,
-3.42584981007467E-5));
#10482=CARTESIAN_POINT('Ctrl Pts',(0.179754261386328,-1.48124444832217,
-3.38986806574493E-5));
#10483=CARTESIAN_POINT('Ctrl Pts',(0.18241086941249,-1.48238102342202,-3.34441145409493E-5));
#10484=CARTESIAN_POINT('Ctrl Pts',(0.199890279181845,-1.48985922935543,
-3.04532527580594E-5));
#10485=CARTESIAN_POINT('Ctrl Pts',(0.217974246898519,-1.49569663469242,
-2.31073027206853E-5));
#10486=CARTESIAN_POINT('Ctrl Pts',(0.236436446036386,-1.49978781870256,
-1.54828395726751E-5));
#10487=CARTESIAN_POINT('Ctrl Pts',(0.253618559172887,-1.50359533838099,
-8.38702246898572E-6));
#10488=CARTESIAN_POINT('Ctrl Pts',(0.271129804961754,-1.50589051664322,
-1.1237837803371E-6));
#10489=CARTESIAN_POINT('Ctrl Pts',(0.288799387895208,-1.50654014509364,
-1.14426782679271E-7));
#10490=CARTESIAN_POINT('Ctrl Pts',(0.290115790923368,-1.5065885431154,-3.92285953074499E-8));
#10491=CARTESIAN_POINT('Ctrl Pts',(0.291433072638222,-1.50662778343727,
-2.32210426557352E-12));
#10492=CARTESIAN_POINT('Ctrl Pts',(0.292751161823634,-1.50665779898694,
2.86229373536173E-17));
#10493=CARTESIAN_POINT('',(0.,-1.5,0.));
#10494=CARTESIAN_POINT('',(0.297857995688647,-1.306435779838,0.));
#10495=CARTESIAN_POINT('Ctrl Pts',(0.200274469199585,-1.20659878095028,
-5.63785129692462E-18));
#10496=CARTESIAN_POINT('Ctrl Pts',(0.200274469233139,-1.21453676310593,
-8.71436967499621E-13));
#10497=CARTESIAN_POINT('Ctrl Pts',(0.201246859971722,-1.22243356087926,
-1.21395871814677E-6));
#10498=CARTESIAN_POINT('Ctrl Pts',(0.203115675186186,-1.23012372049816,
-1.3343733317444E-6));
#10499=CARTESIAN_POINT('Ctrl Pts',(0.204315340901654,-1.23506033529553,
-1.41167219064517E-6));
#10500=CARTESIAN_POINT('Ctrl Pts',(0.20588557457721,-1.23991201018842,-1.08820351238587E-6));
#10501=CARTESIAN_POINT('Ctrl Pts',(0.207817175189242,-1.24463217458037,
-4.7123943162984E-7));
#10502=CARTESIAN_POINT('Ctrl Pts',(0.210821635148072,-1.25197403646754,
4.8840194822981E-7));
#10503=CARTESIAN_POINT('Ctrl Pts',(0.214662962735955,-1.25891288736431,
2.34840446672759E-6));
#10504=CARTESIAN_POINT('Ctrl Pts',(0.219285851586231,-1.26528190572196,
1.77850405974346E-6));
#10505=CARTESIAN_POINT('Ctrl Pts',(0.219987799701267,-1.26624898941694,
1.69196931287913E-6));
#10506=CARTESIAN_POINT('Ctrl Pts',(0.220707854727247,-1.26720289123473,
1.54254180957111E-6));
#10507=CARTESIAN_POINT('Ctrl Pts',(0.221445913570039,-1.26814297034805,
1.31084431541716E-6));
#10508=CARTESIAN_POINT('Ctrl Pts',(0.223819423285066,-1.27116615329633,
5.65732650279818E-7));
#10509=CARTESIAN_POINT('Ctrl Pts',(0.226378993511503,-1.27404655624932,
-1.0141799309673E-6));
#10510=CARTESIAN_POINT('Ctrl Pts',(0.229108317341547,-1.27677508245113,
-2.75886047820546E-6));
#10511=CARTESIAN_POINT('Ctrl Pts',(0.234729699316268,-1.28239482161129,
-6.35224711555937E-6));
#10512=CARTESIAN_POINT('Ctrl Pts',(0.241002345945823,-1.28730653457646,
-1.03364935932408E-5));
#10513=CARTESIAN_POINT('Ctrl Pts',(0.247764463424355,-1.29145035967733,
-1.17765252099068E-5));
#10514=CARTESIAN_POINT('Ctrl Pts',(0.25202072563572,-1.29405859685204,-1.26829206064147E-5));
#10515=CARTESIAN_POINT('Ctrl Pts',(0.25647185453211,-1.29636195369988,-1.26655904667795E-5));
#10516=CARTESIAN_POINT('Ctrl Pts',(0.261083107941716,-1.29833661269995,
-1.17517412599227E-5));
#10517=CARTESIAN_POINT('Ctrl Pts',(0.268362152520619,-1.30145368947124,
-1.0309194402435E-5));
#10518=CARTESIAN_POINT('Ctrl Pts',(0.275955349537693,-1.30371808689536,
-6.50743389458559E-6));
#10519=CARTESIAN_POINT('Ctrl Pts',(0.283717840216357,-1.30505580179168,
-3.40467605837577E-6));
#10520=CARTESIAN_POINT('Ctrl Pts',(0.288379557365255,-1.3058591584372,-1.54133347766382E-6));
#10521=CARTESIAN_POINT('Ctrl Pts',(0.293102847896135,-1.30632748638856,
-3.09915230996644E-12));
#10522=CARTESIAN_POINT('Ctrl Pts',(0.297857995688647,-1.306435779838,2.90566182226115E-17));
#10523=CARTESIAN_POINT('',(0.9,-1.32024227787037,0.));
#10524=CARTESIAN_POINT('Ctrl Pts',(0.297857995688651,-1.306435779838,-5.81335652359571E-17));
#10525=CARTESIAN_POINT('Ctrl Pts',(0.498765834064439,-1.31101124067384,
-1.02216845336465E-13));
#10526=CARTESIAN_POINT('Ctrl Pts',(0.699470314209512,-1.31560060357718,
-4.73070532165219E-10));
#10527=CARTESIAN_POINT('Ctrl Pts',(0.9,-1.32024227787037,4.62320796019307E-17));
#10528=CARTESIAN_POINT('',(0.9,1.39290118819044,0.));
#10529=CARTESIAN_POINT('',(4.3,-1.41116952203211,0.));
#10530=CARTESIAN_POINT('Ctrl Pts',(1.10000000020724,-1.32489175811528,-9.82782277325449E-12));
#10531=CARTESIAN_POINT('Ctrl Pts',(2.16992692797068,-1.34987955410658,4.63225598025733E-9));
#10532=CARTESIAN_POINT('Ctrl Pts',(3.23514201430925,-1.37672428034078,3.20747301048384E-8));
#10533=CARTESIAN_POINT('Ctrl Pts',(4.3,-1.41116952203211,-8.74629427996717E-16));
#10534=CARTESIAN_POINT('',(4.3,1.48481481481482,0.));
#10535=CARTESIAN_POINT('',(8.7,-1.61160179736194,0.));
#10536=CARTESIAN_POINT('Ctrl Pts',(4.50000000001737,-1.41772989873549,-1.00870158580013E-12));
#10537=CARTESIAN_POINT('Ctrl Pts',(5.14541122039116,-1.43919849219739,1.84287460122322E-8));
#10538=CARTESIAN_POINT('Ctrl Pts',(5.79079200637672,-1.46358894290692,-2.29215846350395E-9));
#10539=CARTESIAN_POINT('Ctrl Pts',(6.43711407552466,-1.49221504703413,-7.12038357450289E-9));
#10540=CARTESIAN_POINT('Ctrl Pts',(6.48784335049204,-1.49446188584227,-7.49934689782436E-9));
#10541=CARTESIAN_POINT('Ctrl Pts',(6.5385784252675,-1.49673484630497,-7.6873350528488E-9));
#10542=CARTESIAN_POINT('Ctrl Pts',(6.58931977021612,-1.49903457911226,-7.60400982311631E-9));
#10543=CARTESIAN_POINT('Ctrl Pts',(7.29382172663923,-1.5309644828944,-6.44710735180711E-9));
#10544=CARTESIAN_POINT('Ctrl Pts',(7.99729122590638,-1.56795478022256,5.29179522587699E-9));
#10545=CARTESIAN_POINT('Ctrl Pts',(8.70000000002062,-1.61160179731554,-3.21479112539667E-13));
#10546=CARTESIAN_POINT('',(8.7,1.68851851851852,0.));
#10547=CARTESIAN_POINT('',(12.6,-1.93292824674167,0.));
#10548=CARTESIAN_POINT('',(12.8889963716306,-1.96391015057091,0.));
#10549=CARTESIAN_POINT('Ctrl Pts',(12.6000000004653,-1.93292824679067,-1.00288700954909E-16));
#10550=CARTESIAN_POINT('Ctrl Pts',(12.6963367945484,-1.94307238002033,2.28133307867826E-10));
#10551=CARTESIAN_POINT('Ctrl Pts',(12.7926686848896,-1.9533982851754,-5.07154825701885E-13));
#10552=CARTESIAN_POINT('Ctrl Pts',(12.8889963716306,-1.96391015057091,2.24786696790336E-16));
#10553=CARTESIAN_POINT('',(12.9997255308004,-1.86463850151065,-1.38777878078145E-17));
#10554=CARTESIAN_POINT('Ctrl Pts',(12.8889963716306,-1.96391015057091,5.29090660172926E-17));
#10555=CARTESIAN_POINT('Ctrl Pts',(12.8968843421745,-1.96477093437063,1.28387508960266E-11));
#10556=CARTESIAN_POINT('Ctrl Pts',(12.9048206871516,-1.96464841285931,-2.5989605143924E-6));
#10557=CARTESIAN_POINT('Ctrl Pts',(12.9126487282508,-1.9636130141884,-4.24292438262167E-6));
#10558=CARTESIAN_POINT('Ctrl Pts',(12.9176900487482,-1.96294620923983,-5.30165014054907E-6));
#10559=CARTESIAN_POINT('Ctrl Pts',(12.9226867577298,-1.96189962975099,-6.00943773338864E-6));
#10560=CARTESIAN_POINT('Ctrl Pts',(12.9275953864907,-1.96048085896027,-6.09358828708331E-6));
#10561=CARTESIAN_POINT('Ctrl Pts',(12.9352257743335,-1.95827540160737,-6.22439902734509E-6));
#10562=CARTESIAN_POINT('Ctrl Pts',(12.9425549137553,-1.95519874430406,-4.64402662178521E-6));
#10563=CARTESIAN_POINT('Ctrl Pts',(12.949425376669,-1.9513005478593,-3.15156624759025E-6));
#10564=CARTESIAN_POINT('Ctrl Pts',(12.9520760960011,-1.94979656991686,-2.57575445499556E-6));
#10565=CARTESIAN_POINT('Ctrl Pts',(12.9546583803074,-1.94816978416017,-2.04880625960079E-6));
#10566=CARTESIAN_POINT('Ctrl Pts',(12.9571622133441,-1.9464211898676,-1.82278374303809E-6));
#10567=CARTESIAN_POINT('Ctrl Pts',(12.9587955877505,-1.9452804951316,-1.67533805140214E-6));
#10568=CARTESIAN_POINT('Ctrl Pts',(12.9603955609302,-1.94408794089591,-1.65796127395168E-6));
#10569=CARTESIAN_POINT('Ctrl Pts',(12.9619602112942,-1.94284549575182,-1.70649031798611E-6));
#10570=CARTESIAN_POINT('Ctrl Pts',(12.9681665721336,-1.93791719798967,-1.89898620422551E-6));
#10571=CARTESIAN_POINT('Ctrl Pts',(12.9737470546445,-1.93226498850035,-2.8025064238469E-6));
#10572=CARTESIAN_POINT('Ctrl Pts',(12.9786034821464,-1.926037248212,-2.79230211737029E-6));
#10573=CARTESIAN_POINT('Ctrl Pts',(12.9817011960737,-1.92206483066456,-2.78579321297956E-6));
#10574=CARTESIAN_POINT('Ctrl Pts',(12.9845038017717,-1.91785723501915,-2.48811564693169E-6));
#10575=CARTESIAN_POINT('Ctrl Pts',(12.9869771252785,-1.91344616543364,-2.2918341012218E-6));
#10576=CARTESIAN_POINT('Ctrl Pts',(12.9874796596041,-1.91254991636901,-2.25195326317628E-6));
#10577=CARTESIAN_POINT('Ctrl Pts',(12.9879679417815,-1.9116463809131,-2.21866365029432E-6));
#10578=CARTESIAN_POINT('Ctrl Pts',(12.98844174868,-1.91073586520696,-2.19841011183313E-6));
#10579=CARTESIAN_POINT('Ctrl Pts',(12.9918929665356,-1.9041036526468,-2.05088297829219E-6));
#10580=CARTESIAN_POINT('Ctrl Pts',(12.9945793344589,-1.89710244289626,-2.35789128083535E-6));
#10581=CARTESIAN_POINT('Ctrl Pts',(12.9964698429198,-1.88986530397042,-1.93853625224654E-6));
#10582=CARTESIAN_POINT('Ctrl Pts',(12.9984668213505,-1.88222058265133,-1.49556391743615E-6));
#10583=CARTESIAN_POINT('Ctrl Pts',(12.9995610814633,-1.87437060764114,-2.4459616079733E-7));
#10584=CARTESIAN_POINT('Ctrl Pts',(12.9997084424383,-1.86646992060833,-2.60951667192209E-8));
#10585=CARTESIAN_POINT('Ctrl Pts',(12.9997198235207,-1.86585972940924,-9.21975031242219E-9));
#10586=CARTESIAN_POINT('Ctrl Pts',(12.9997255308031,-1.86524923282631,2.14479566203628E-13));
#10587=CARTESIAN_POINT('Ctrl Pts',(12.9997255308004,-1.86463850151065,-9.54097911787244E-18));
#10588=CARTESIAN_POINT('',(12.9997255308004,1.86463850151064,1.38777878078145E-17));
#10589=CARTESIAN_POINT('',(12.9997255308004,1.1,0.));
#10590=CARTESIAN_POINT('',(12.8889963716306,1.96391015057091,0.));
#10591=CARTESIAN_POINT('Ctrl Pts',(12.9997255308004,1.86463850151065,-9.97465998686664E-18));
#10592=CARTESIAN_POINT('Ctrl Pts',(12.9997255309996,1.87257112921612,1.42345874390777E-11));
#10593=CARTESIAN_POINT('Ctrl Pts',(12.9987425107347,1.88044501776258,-2.76622459581243E-6));
#10594=CARTESIAN_POINT('Ctrl Pts',(12.9968635501128,1.8881121101061,-4.50602169498049E-6));
#10595=CARTESIAN_POINT('Ctrl Pts',(12.9956551765012,1.89304287446485,-5.62489820561454E-6));
#10596=CARTESIAN_POINT('Ctrl Pts',(12.994075066483,1.89788828888188,-6.37205869803057E-6));
#10597=CARTESIAN_POINT('Ctrl Pts',(12.9921354490207,1.90260616696402,-6.45954116508302E-6));
#10598=CARTESIAN_POINT('Ctrl Pts',(12.9891151690915,1.90995262200289,-6.59576469602218E-6));
#10599=CARTESIAN_POINT('Ctrl Pts',(12.9852608829945,1.91690476599405,-4.92589918404109E-6));
#10600=CARTESIAN_POINT('Ctrl Pts',(12.9806393828366,1.92331154882078,-3.3382766296878E-6));
#10601=CARTESIAN_POINT('Ctrl Pts',(12.9788533632605,1.92578750666072,-2.72472586378502E-6));
#10602=CARTESIAN_POINT('Ctrl Pts',(12.9769522584487,1.92818179997524,-2.1610482659023E-6));
#10603=CARTESIAN_POINT('Ctrl Pts',(12.9749381758772,1.93048453804291,-1.90960564360578E-6));
#10604=CARTESIAN_POINT('Ctrl Pts',(12.9736352090466,1.93197424425657,-1.74694031832382E-6));
#10605=CARTESIAN_POINT('Ctrl Pts',(12.9722849384098,1.93342561524533,-1.71698229815602E-6));
#10606=CARTESIAN_POINT('Ctrl Pts',(12.9708894910408,1.9348369915754,-1.75552529092739E-6));
#10607=CARTESIAN_POINT('Ctrl Pts',(12.9653179015399,1.94047218048862,-1.90941553332435E-6));
#10608=CARTESIAN_POINT('Ctrl Pts',(12.9590944588136,1.94540670303376,-2.83773366290493E-6));
#10609=CARTESIAN_POINT('Ctrl Pts',(12.9523775255978,1.94955941520082,-2.8574013135715E-6));
#10610=CARTESIAN_POINT('Ctrl Pts',(12.9480923984168,1.95220867479748,-2.86994846593266E-6));
#10611=CARTESIAN_POINT('Ctrl Pts',(12.9436054681019,1.95453912223498,-2.59559485065602E-6));
#10612=CARTESIAN_POINT('Ctrl Pts',(12.9389519978263,1.95652032281755,-2.39773084743613E-6));
#10613=CARTESIAN_POINT('Ctrl Pts',(12.9379934875219,1.95692840561619,-2.35697530915642E-6));
#10614=CARTESIAN_POINT('Ctrl Pts',(12.9370291206935,1.95732112306527,-2.32193094846859E-6));
#10615=CARTESIAN_POINT('Ctrl Pts',(12.9360592398442,1.95769827921557,-2.29894501965994E-6));
#10616=CARTESIAN_POINT('Ctrl Pts',(12.929096105975,1.96040602292032,-2.13392052256244E-6));
#10617=CARTESIAN_POINT('Ctrl Pts',(12.9218497638689,1.96231496375013,-2.36509085467933E-6));
#10618=CARTESIAN_POINT('Ctrl Pts',(12.9144555496645,1.96340894166242,-1.92146179377921E-6));
#10619=CARTESIAN_POINT('Ctrl Pts',(12.9066371708262,1.96456567495722,-1.45238421961943E-6));
#10620=CARTESIAN_POINT('Ctrl Pts',(12.8987125532455,1.96480297730229,-2.37321368026999E-7));
#10621=CARTESIAN_POINT('Ctrl Pts',(12.8908401755085,1.96409377829808,-2.55627471131237E-8));
#10622=CARTESIAN_POINT('Ctrl Pts',(12.89022523009,1.96403837970149,-9.02136684357828E-9));
#10623=CARTESIAN_POINT('Ctrl Pts',(12.8896106033158,1.96397717928728,1.9621770460073E-13));
#10624=CARTESIAN_POINT('Ctrl Pts',(12.8889963716306,1.96391015057091,-3.29597460435593E-17));
#10625=CARTESIAN_POINT('',(12.6,1.93292824674167,0.));
#10626=CARTESIAN_POINT('Ctrl Pts',(12.8889963716306,1.96391015057091,8.95144418658345E-17));
#10627=CARTESIAN_POINT('Ctrl Pts',(12.7926686852738,1.95339828521733,-5.07275478770449E-13));
#10628=CARTESIAN_POINT('Ctrl Pts',(12.6963367949308,1.94307238006059,2.28132759158623E-10));
#10629=CARTESIAN_POINT('Ctrl Pts',(12.6000000004652,1.93292824679066,-1.5019386425618E-16));
#10630=CARTESIAN_POINT('',(12.6,-1.99376954809806,0.));
#10631=CARTESIAN_POINT('Origin',(11.2,0.,0.));
#10632=CARTESIAN_POINT('',(10.8,-4.89858719658942E-17,0.7));
#10633=CARTESIAN_POINT('Origin',(11.2,0.,0.7));
#10634=CARTESIAN_POINT('',(10.8,-4.89858719658942E-17,0.));
#10635=CARTESIAN_POINT('Origin',(2.,0.,0.));
#10636=CARTESIAN_POINT('',(1.6,-4.89858719658941E-17,0.));
#10637=CARTESIAN_POINT('Origin',(12.6,-1.99376954809806,0.));
#10638=CARTESIAN_POINT('',(12.6,-1.90428042248893,0.60470250816874));
#10639=CARTESIAN_POINT('Ctrl Pts',(12.6,-1.93292824674167,0.));
#10640=CARTESIAN_POINT('Ctrl Pts',(12.6,-1.92814118331811,0.100975624959503));
#10641=CARTESIAN_POINT('Ctrl Pts',(12.6,-1.9233557423333,0.20195205683881));
#10642=CARTESIAN_POINT('Ctrl Pts',(12.6,-1.91380649287245,0.40351907263528));
#10643=CARTESIAN_POINT('Ctrl Pts',(12.6,-1.90904260275794,0.504111110768618));
#10644=CARTESIAN_POINT('Ctrl Pts',(12.6,-1.90428042248893,0.60470250816874));
#10645=CARTESIAN_POINT('',(12.6,1.90428042248893,0.60470250816874));
#10646=CARTESIAN_POINT('Ctrl Pts',(12.6,1.90428042248893,0.60470250816874));
#10647=CARTESIAN_POINT('Ctrl Pts',(12.6,1.90904310126474,0.504100580823831));
#10648=CARTESIAN_POINT('Ctrl Pts',(12.6,1.91380749024866,0.403498012513773));
#10649=CARTESIAN_POINT('Ctrl Pts',(12.6,1.92335674041114,0.201930996640285));
#10650=CARTESIAN_POINT('Ctrl Pts',(12.6,1.92814168252712,0.100965094925255));
#10651=CARTESIAN_POINT('Ctrl Pts',(12.6,1.93292824674167,0.));
#10652=CARTESIAN_POINT('',(12.6,1.80383022254432,0.7));
#10653=CARTESIAN_POINT('Ctrl Pts',(12.6,1.80383022254432,0.7));
#10654=CARTESIAN_POINT('Ctrl Pts',(12.6,1.81177675668304,0.7));
#10655=CARTESIAN_POINT('Ctrl Pts',(12.6000021803669,1.81966206665253,0.699006623620781));
#10656=CARTESIAN_POINT('Ctrl Pts',(12.6000040789681,1.8273451885609,0.69711902809518));
#10657=CARTESIAN_POINT('Ctrl Pts',(12.6000050614635,1.8313210797205,0.696142227980247));
#10658=CARTESIAN_POINT('Ctrl Pts',(12.6000059683507,1.83524283435206,0.694925046992878));
#10659=CARTESIAN_POINT('Ctrl Pts',(12.6000066021136,1.83908960013903,0.693475985595303));
#10660=CARTESIAN_POINT('Ctrl Pts',(12.6000078338507,1.84656590463324,0.690659691378536));
#10661=CARTESIAN_POINT('Ctrl Pts',(12.6000078244032,1.85367932786264,0.687000939374075));
#10662=CARTESIAN_POINT('Ctrl Pts',(12.6000065509639,1.86028396908448,0.682580904467878));
#10663=CARTESIAN_POINT('Ctrl Pts',(12.600005740321,1.86448833536622,0.679767209507086));
#10664=CARTESIAN_POINT('Ctrl Pts',(12.6000044390918,1.86848632867783,0.676643963831362));
#10665=CARTESIAN_POINT('Ctrl Pts',(12.6000033339006,1.8722338275817,0.673223162566374));
#10666=CARTESIAN_POINT('Ctrl Pts',(12.6000024442799,1.87525036668517,0.670469597843409));
#10667=CARTESIAN_POINT('Ctrl Pts',(12.600001679327,1.8780865799519,0.667539409933064));
#10668=CARTESIAN_POINT('Ctrl Pts',(12.600001676908,1.88072259809992,0.664442334323256));
#10669=CARTESIAN_POINT('Ctrl Pts',(12.6000016722164,1.88583495965423,0.658435786041233));
#10670=CARTESIAN_POINT('Ctrl Pts',(12.6000042182276,1.89019731592974,0.651802923597933));
#10671=CARTESIAN_POINT('Ctrl Pts',(12.6000050838539,1.89374834224248,0.644708005294394));
#10672=CARTESIAN_POINT('Ctrl Pts',(12.60000518898,1.89417959722901,0.643846361750254));
#10673=CARTESIAN_POINT('Ctrl Pts',(12.6000052753339,1.8945988291305,0.642977876839351));
#10674=CARTESIAN_POINT('Ctrl Pts',(12.6000053405091,1.89500587920016,0.642102827114796));
#10675=CARTESIAN_POINT('Ctrl Pts',(12.6000058761205,1.89835102950234,0.634911640898031));
#10676=CARTESIAN_POINT('Ctrl Pts',(12.6000044960414,1.90083797337412,0.627363460372113));
#10677=CARTESIAN_POINT('Ctrl Pts',(12.6000025707297,1.90241244660326,0.619625605651968));
#10678=CARTESIAN_POINT('Ctrl Pts',(12.6000013488022,1.90341170938816,0.614714661398562));
#10679=CARTESIAN_POINT('Ctrl Pts',(12.5999999979477,1.90404256918024,0.609726685483646));
#10680=CARTESIAN_POINT('Ctrl Pts',(12.6000000000242,1.90428042250026,0.604702508168697));
#10681=CARTESIAN_POINT('',(12.6,-1.8038302225439,0.7));
#10682=CARTESIAN_POINT('',(12.6,-0.996884774049031,0.7));
#10683=CARTESIAN_POINT('Ctrl Pts',(12.6000000000242,-1.90428042250026,0.604702508168697));
#10684=CARTESIAN_POINT('Ctrl Pts',(12.5999999967566,-1.90390613686288,0.612608546261599));
#10685=CARTESIAN_POINT('Ctrl Pts',(12.6000030637542,-1.90256112855112,0.620429349781532));
#10686=CARTESIAN_POINT('Ctrl Pts',(12.6000044618611,-1.90032851942705,0.628004813168584));
#10687=CARTESIAN_POINT('Ctrl Pts',(12.6000051410147,-1.89924399238468,0.63168472059761));
#10688=CARTESIAN_POINT('Ctrl Pts',(12.6000055125137,-1.89794920179963,0.635306724151721));
#10689=CARTESIAN_POINT('Ctrl Pts',(12.6000054780251,-1.8964494555225,0.638851301608537));
#10690=CARTESIAN_POINT('Ctrl Pts',(12.6000054068101,-1.89335265044601,0.64617044994032));
#10691=CARTESIAN_POINT('Ctrl Pts',(12.6000033360581,-1.88942004582711,0.653077891556402));
#10692=CARTESIAN_POINT('Ctrl Pts',(12.6000021947065,-1.88472046879005,0.659412676045522));
#10693=CARTESIAN_POINT('Ctrl Pts',(12.6000018847951,-1.88344439178375,0.661132761228218));
#10694=CARTESIAN_POINT('Ctrl Pts',(12.6000016718208,-1.88211149822114,0.662810505670431));
#10695=CARTESIAN_POINT('Ctrl Pts',(12.6000016744967,-1.88072259784382,0.664442334323417));
#10696=CARTESIAN_POINT('Ctrl Pts',(12.6000016781594,-1.87882150924004,0.666675936463772));
#10697=CARTESIAN_POINT('Ctrl Pts',(12.6000020841502,-1.87681550570489,0.668823545630641));
#10698=CARTESIAN_POINT('Ctrl Pts',(12.6000026366798,-1.87471194035196,0.670881441794774));
#10699=CARTESIAN_POINT('Ctrl Pts',(12.6000041308351,-1.86902346102148,0.676446422116204));
#10700=CARTESIAN_POINT('Ctrl Pts',(12.600006461375,-1.86269053299793,0.681293522350018));
#10701=CARTESIAN_POINT('Ctrl Pts',(12.6000072160154,-1.85587841208407,0.685370830723365));
#10702=CARTESIAN_POINT('Ctrl Pts',(12.6000077023835,-1.85148797774957,0.687998669380522));
#10703=CARTESIAN_POINT('Ctrl Pts',(12.6000076405209,-1.84689749427555,0.690306084934615));
#10704=CARTESIAN_POINT('Ctrl Pts',(12.6000070464578,-1.84214500723865,0.692269637845719));
#10705=CARTESIAN_POINT('Ctrl Pts',(12.6000061272438,-1.8347913233911,0.69530790964196));
#10706=CARTESIAN_POINT('Ctrl Pts',(12.6000039197963,-1.82713360831075,0.697490862850871));
#10707=CARTESIAN_POINT('Ctrl Pts',(12.6000021173902,-1.81932000848244,0.698749700991972));
#10708=CARTESIAN_POINT('Ctrl Pts',(12.6000009388424,-1.81421089282246,0.699572823470905));
#10709=CARTESIAN_POINT('Ctrl Pts',(12.6,-1.80903450780073,0.7));
#10710=CARTESIAN_POINT('Ctrl Pts',(12.6,-1.80383022254432,0.7));
#10711=CARTESIAN_POINT('Ctrl Pts',(12.4277899437912,-1.91498765980368,8.1061082099175E-6));
#10712=CARTESIAN_POINT('Ctrl Pts',(12.4185093097394,-1.90440735427916,0.201956437811591));
#10713=CARTESIAN_POINT('Ctrl Pts',(12.4092288296506,-1.89382707230216,0.403904777849331));
#10714=CARTESIAN_POINT('Ctrl Pts',(12.3999485057213,-1.88324681432718,0.605853126346544));
#10715=CARTESIAN_POINT('Ctrl Pts',(11.2514531524596,-1.79377193015415,-0.000335869645892519));
#10716=CARTESIAN_POINT('Ctrl Pts',(11.2440495594319,-1.78319067664719,0.201611894978303));
#10717=CARTESIAN_POINT('Ctrl Pts',(11.2366461029568,-1.77260943823668,0.403559665746509));
#10718=CARTESIAN_POINT('Ctrl Pts',(11.2292427771396,-1.76202821861547,0.605507441576721));
#10719=CARTESIAN_POINT('Ctrl Pts',(10.0755218259154,-1.69940246002113,-0.00057195363688788));
#10720=CARTESIAN_POINT('Ctrl Pts',(10.0699958446785,-1.68882059084335,0.201375418496625));
#10721=CARTESIAN_POINT('Ctrl Pts',(10.0644699805481,-1.67823873210945,0.403322794723726));
#10722=CARTESIAN_POINT('Ctrl Pts',(10.0589442279885,-1.66765688783508,0.605270174140068));
#10723=CARTESIAN_POINT('Ctrl Pts',(8.90001330805802,-1.62424530699552,-0.000736768987564917));
#10724=CARTESIAN_POINT('Ctrl Pts',(8.89636559238287,-1.61366301035882,0.201210329036737));
#10725=CARTESIAN_POINT('Ctrl Pts',(8.89271797406169,-1.60308072296431,0.403157429313698));
#10726=CARTESIAN_POINT('Ctrl Pts',(8.88907045450167,-1.59249844499155,0.605104531878289));
#10727=CARTESIAN_POINT('Ctrl Pts',(8.9000000009702,-1.5932011715731,0.605106081469384));
#10728=CARTESIAN_POINT('Ctrl Pts',(10.0684994345535,-1.66840362346204,0.605023135335662));
#10729=CARTESIAN_POINT('Ctrl Pts',(11.2356615742313,-1.76272273105624,0.604904457271936));
#10730=CARTESIAN_POINT('Ctrl Pts',(12.4,-1.8833055216247,0.604732563714112));
#10731=CARTESIAN_POINT('Ctrl Pts',(12.8889963716306,-1.96391015057091,2.25514051876985E-16));
#10732=CARTESIAN_POINT('Ctrl Pts',(12.8789974396847,-1.95334878321431,0.201594505485581));
#10733=CARTESIAN_POINT('Ctrl Pts',(12.8689986695879,-1.94278744208821,0.403189020401051));
#10734=CARTESIAN_POINT('Ctrl Pts',(12.8590000636394,-1.93222612769726,0.604783544887274));
#10735=CARTESIAN_POINT('Ctrl Pts',(12.792662965057,-1.95339909479377,-3.05216148415599E-5));
#10736=CARTESIAN_POINT('Ctrl Pts',(12.7828174539371,-1.94283764251598,0.201563933758495));
#10737=CARTESIAN_POINT('Ctrl Pts',(12.7729721028852,-1.93227621586528,0.403158398317997));
#10738=CARTESIAN_POINT('Ctrl Pts',(12.7631269141758,-1.92171481533493,0.604752872200892));
#10739=CARTESIAN_POINT('Ctrl Pts',(12.6963322449993,-1.94307475200589,-6.02899321993968E-5));
#10740=CARTESIAN_POINT('Ctrl Pts',(12.6866401583647,-1.93251321719056,0.201534116532542));
#10741=CARTESIAN_POINT('Ctrl Pts',(12.6769482300299,-1.92195170741534,0.403128531945268));
#10742=CARTESIAN_POINT('Ctrl Pts',(12.6672564622455,-1.91139022316239,0.604722956439736));
#10743=CARTESIAN_POINT('Ctrl Pts',(12.6000042264769,-1.9329329264796,-8.93242901516475E-5));
#10744=CARTESIAN_POINT('Ctrl Pts',(12.5904655680581,-1.92237131142302,0.201505034443145));
#10745=CARTESIAN_POINT('Ctrl Pts',(12.5809270661843,-1.91180972083551,0.403099401891705));
#10746=CARTESIAN_POINT('Ctrl Pts',(12.5713887230828,-1.90124815518829,0.604693778185974));
#10747=CARTESIAN_POINT('',(12.8572578715866,-1.93204080633595,0.60466226999893));
#10748=CARTESIAN_POINT('Ctrl Pts',(12.6000000000242,-1.90428042250026,0.604702508168697));
#10749=CARTESIAN_POINT('Ctrl Pts',(12.6857696261193,-1.91338852735451,0.604689390578107));
#10750=CARTESIAN_POINT('Ctrl Pts',(12.7715225733429,-1.92264108900731,0.604675979983877));
#10751=CARTESIAN_POINT('Ctrl Pts',(12.8572578715866,-1.93204080633595,0.60466226999893));
#10752=CARTESIAN_POINT('Ctrl Pts',(12.8572578715866,-1.93204080633595,0.604662269998931));
#10753=CARTESIAN_POINT('Ctrl Pts',(12.867837444884,-1.94266422047353,0.403108198925376));
#10754=CARTESIAN_POINT('Ctrl Pts',(12.8784169445746,-1.95328733374019,0.201554108835025));
#10755=CARTESIAN_POINT('Ctrl Pts',(12.8889963716306,-1.96391015057091,-1.13624387676481E-16));
#10756=CARTESIAN_POINT('Ctrl Pts',(12.4102890066107,-1.7839488953552,0.7));
#10757=CARTESIAN_POINT('Ctrl Pts',(11.2423261062923,-1.6629989551888,0.7));
#10758=CARTESIAN_POINT('Ctrl Pts',(10.0717272052363,-1.56846077660453,0.7));
#10759=CARTESIAN_POINT('Ctrl Pts',(8.89999999999993,-1.49312521822106,0.7));
#10760=CARTESIAN_POINT('Ctrl Pts',(12.4072999778185,-1.81281269415102,0.7));
#10761=CARTESIAN_POINT('Ctrl Pts',(11.2397765858669,-1.69187462084457,0.699998757165067));
#10762=CARTESIAN_POINT('Ctrl Pts',(10.0695527221263,-1.59734372851255,0.700000594792869));
#10763=CARTESIAN_POINT('Ctrl Pts',(8.89814271406455,-1.52201240649035,0.7));
#10764=CARTESIAN_POINT('Ctrl Pts',(12.4021203845267,-1.86282985658401,0.676448561733929));
#10765=CARTESIAN_POINT('Ctrl Pts',(11.2353531757414,-1.74191593276004,0.676505236381959));
#10766=CARTESIAN_POINT('Ctrl Pts',(10.0657879841113,-1.64739716848489,0.676543604639643));
#10767=CARTESIAN_POINT('Ctrl Pts',(8.89492397206972,-1.57207492202614,0.676570833338327));
#10768=CARTESIAN_POINT('Ctrl Pts',(12.400106093269,-1.88228102337346,0.626471792264191));
#10769=CARTESIAN_POINT('Ctrl Pts',(11.2336287644773,-1.76143987438699,0.626617923584012));
#10770=CARTESIAN_POINT('Ctrl Pts',(10.0643137348541,-1.66697079985262,0.626717999675944));
#10771=CARTESIAN_POINT('Ctrl Pts',(8.89366330605793,-1.59168261717615,0.626788336025017));
#10772=CARTESIAN_POINT('Ctrl Pts',(12.4,-1.8833055216247,0.604732563714112));
#10773=CARTESIAN_POINT('Ctrl Pts',(11.2335332423564,-1.7625023138725,0.604904771481731));
#10774=CARTESIAN_POINT('Ctrl Pts',(10.0642324382527,-1.66805889332185,0.605023569028795));
#10775=CARTESIAN_POINT('Ctrl Pts',(8.89359217382714,-1.59278896817116,0.605106535971077));
#10776=CARTESIAN_POINT('Ctrl Pts',(12.400000003046,-1.78288409409898,0.7));
#10777=CARTESIAN_POINT('Ctrl Pts',(11.235451325406,-1.66244391065713,0.7));
#10778=CARTESIAN_POINT('Ctrl Pts',(10.0682865064676,-1.56823955876321,0.7));
#10779=CARTESIAN_POINT('Ctrl Pts',(8.89999999999993,-1.49312521822106,0.7));
#10780=CARTESIAN_POINT('Ctrl Pts',(12.8681436286308,-1.83274446434879,0.7));
#10781=CARTESIAN_POINT('Ctrl Pts',(12.7787800350189,-1.82294762441299,0.7));
#10782=CARTESIAN_POINT('Ctrl Pts',(12.6893984576578,-1.8133105623702,0.7));
#10783=CARTESIAN_POINT('Ctrl Pts',(12.6,-1.80383022254431,0.7));
#10784=CARTESIAN_POINT('Ctrl Pts',(12.8649798835675,-1.86160311979107,0.7));
#10785=CARTESIAN_POINT('Ctrl Pts',(12.7756511334299,-1.85180730951691,0.699999896874207));
#10786=CARTESIAN_POINT('Ctrl Pts',(12.686303642571,-1.84217134991284,0.700000098415946));
#10787=CARTESIAN_POINT('Ctrl Pts',(12.5969393303221,-1.83269196733649,0.7));
#10788=CARTESIAN_POINT('Ctrl Pts',(12.8594976525144,-1.91161025179704,0.676425356750174));
#10789=CARTESIAN_POINT('Ctrl Pts',(12.7702288461641,-1.90181652272411,0.676430055978541));
#10790=CARTESIAN_POINT('Ctrl Pts',(12.6809412203008,-1.89218243450198,0.676434576658958));
#10791=CARTESIAN_POINT('Ctrl Pts',(12.5916356538948,-1.88270499442535,0.67643906321291));
#10792=CARTESIAN_POINT('Ctrl Pts',(12.8573684983393,-1.93103170500986,0.626412260100396));
#10793=CARTESIAN_POINT('Ctrl Pts',(12.7681225846323,-1.92124403769089,0.626424372515079));
#10794=CARTESIAN_POINT('Ctrl Pts',(12.6788572782757,-1.91161594713487,0.626436135819418));
#10795=CARTESIAN_POINT('Ctrl Pts',(12.5895741974899,-1.90214427893475,0.626447702441804));
#10796=CARTESIAN_POINT('Ctrl Pts',(12.8572578715866,-1.93204080633595,0.60466226999893));
#10797=CARTESIAN_POINT('Ctrl Pts',(12.7680127446979,-1.92225628370762,0.604676541242762));
#10798=CARTESIAN_POINT('Ctrl Pts',(12.6787484942245,-1.91263121188365,0.60469048808123));
#10799=CARTESIAN_POINT('Ctrl Pts',(12.5894662143615,-1.9031625467727,0.604704117718382));
#10800=CARTESIAN_POINT('',(12.8681436286308,-1.83274446434879,0.7));
#10801=CARTESIAN_POINT('Ctrl Pts',(12.8681436286308,-1.83274446434879,0.7));
#10802=CARTESIAN_POINT('Ctrl Pts',(12.7787800350189,-1.82294762441299,0.7));
#10803=CARTESIAN_POINT('Ctrl Pts',(12.6893984576578,-1.8133105623702,0.7));
#10804=CARTESIAN_POINT('Ctrl Pts',(12.6,-1.80383022254431,0.7));
#10805=CARTESIAN_POINT('Origin',(12.8681436286308,-1.83274446434879,0.6));
#10806=CARTESIAN_POINT('Origin',(6.87409734069396,-2.22251806091942E-16,
0.7));
#10807=CARTESIAN_POINT('Ctrl Pts',(8.9,1.49312521822106,0.7));
#10808=CARTESIAN_POINT('Ctrl Pts',(10.0682865064677,1.56823955876321,0.7));
#10809=CARTESIAN_POINT('Ctrl Pts',(11.2354513254061,1.66244391065714,0.7));
#10810=CARTESIAN_POINT('Ctrl Pts',(12.4000000030461,1.78288409409899,0.7));
#10811=CARTESIAN_POINT('Origin',(6.87409734069396,-2.22251806091942E-16,
0.7));
#10812=CARTESIAN_POINT('',(12.8681436286308,1.83274446434879,0.7));
#10813=CARTESIAN_POINT('Ctrl Pts',(12.6,1.80383022254432,0.7));
#10814=CARTESIAN_POINT('Ctrl Pts',(12.6893984576578,1.8133105623702,0.7));
#10815=CARTESIAN_POINT('Ctrl Pts',(12.7787800350189,1.82294762441299,0.7));
#10816=CARTESIAN_POINT('Ctrl Pts',(12.8681436286308,1.83274446434879,0.7));
#10817=CARTESIAN_POINT('',(12.8681436286308,1.1,0.7));
#10818=CARTESIAN_POINT('Ctrl Pts',(8.9,1.49312521822106,0.7));
#10819=CARTESIAN_POINT('Ctrl Pts',(10.0717272052363,1.56846077660453,0.7));
#10820=CARTESIAN_POINT('Ctrl Pts',(11.2423261062923,1.6629989551888,0.7));
#10821=CARTESIAN_POINT('Ctrl Pts',(12.4102890066107,1.7839488953552,0.7));
#10822=CARTESIAN_POINT('Ctrl Pts',(8.89814271406461,1.52201240649035,0.7));
#10823=CARTESIAN_POINT('Ctrl Pts',(10.0695527221263,1.59734372851256,0.700000594792869));
#10824=CARTESIAN_POINT('Ctrl Pts',(11.2397765858669,1.69187462084457,0.699998757165067));
#10825=CARTESIAN_POINT('Ctrl Pts',(12.4072999778185,1.81281269415102,0.7));
#10826=CARTESIAN_POINT('Ctrl Pts',(8.89492397206979,1.57207492202615,0.676570833338327));
#10827=CARTESIAN_POINT('Ctrl Pts',(10.0657879841114,1.64739716848489,0.676543604639644));
#10828=CARTESIAN_POINT('Ctrl Pts',(11.2353531757414,1.74191593276004,0.676505236381959));
#10829=CARTESIAN_POINT('Ctrl Pts',(12.4021203845267,1.86282985658401,0.676448561733929));
#10830=CARTESIAN_POINT('Ctrl Pts',(8.89366330605799,1.59168261717616,0.626788336025017));
#10831=CARTESIAN_POINT('Ctrl Pts',(10.0643137348542,1.66697079985262,0.626717999675944));
#10832=CARTESIAN_POINT('Ctrl Pts',(11.2336287644773,1.761439874387,0.626617923584012));
#10833=CARTESIAN_POINT('Ctrl Pts',(12.400106093269,1.88228102337346,0.626471792264191));
#10834=CARTESIAN_POINT('Ctrl Pts',(8.89359217382721,1.59278896817116,0.605106535971077));
#10835=CARTESIAN_POINT('Ctrl Pts',(10.0642324382527,1.66805889332185,0.605023569028795));
#10836=CARTESIAN_POINT('Ctrl Pts',(11.2335332423565,1.7625023138725,0.604904771481731));
#10837=CARTESIAN_POINT('Ctrl Pts',(12.4,1.8833055216247,0.604732563714112));
#10838=CARTESIAN_POINT('Ctrl Pts',(12.4,1.8833055216247,0.604732563714112));
#10839=CARTESIAN_POINT('Ctrl Pts',(11.2356615742313,1.76272273105624,0.604904457271936));
#10840=CARTESIAN_POINT('Ctrl Pts',(10.0684994345535,1.66840362346204,0.605023135335662));
#10841=CARTESIAN_POINT('Ctrl Pts',(8.90000000097019,1.5932011715731,0.605106081469384));
#10842=CARTESIAN_POINT('Ctrl Pts',(8.90001330805765,1.62424530699444,-0.000736768966955875));
#10843=CARTESIAN_POINT('Ctrl Pts',(8.89636559238262,1.6136630103581,0.201210329050476));
#10844=CARTESIAN_POINT('Ctrl Pts',(8.89271797406156,1.60308072296395,0.403157429320568));
#10845=CARTESIAN_POINT('Ctrl Pts',(8.88907045450167,1.59249844499155,0.605104531878289));
#10846=CARTESIAN_POINT('Ctrl Pts',(10.0755218259151,1.69940246002007,-0.000571953616278766));
#10847=CARTESIAN_POINT('Ctrl Pts',(10.0699958446785,1.68882059084265,0.201375418510364));
#10848=CARTESIAN_POINT('Ctrl Pts',(10.0644699805483,1.67823873210911,0.403322794730596));
#10849=CARTESIAN_POINT('Ctrl Pts',(10.0589442279888,1.6676568878351,0.605270174140069));
#10850=CARTESIAN_POINT('Ctrl Pts',(11.2514531524595,1.79377193015312,-0.000335869625283423));
#10851=CARTESIAN_POINT('Ctrl Pts',(11.244049559432,1.78319067664652,0.201611894992042));
#10852=CARTESIAN_POINT('Ctrl Pts',(11.2366461029572,1.77260943823637,0.403559665753379));
#10853=CARTESIAN_POINT('Ctrl Pts',(11.2292427771402,1.76202821861552,0.605507441576721));
#10854=CARTESIAN_POINT('Ctrl Pts',(12.4277899437912,1.9149876598027,8.10612881915578E-6));
#10855=CARTESIAN_POINT('Ctrl Pts',(12.4185093097397,1.90440735427854,0.201956437825331));
#10856=CARTESIAN_POINT('Ctrl Pts',(12.4092288296513,1.89382707230189,0.403904777856201));
#10857=CARTESIAN_POINT('Ctrl Pts',(12.3999485057223,1.88324681432728,0.605853126346545));
#10858=CARTESIAN_POINT('Ctrl Pts',(12.6000042264759,1.9329329264795,-8.93242901520291E-5));
#10859=CARTESIAN_POINT('Ctrl Pts',(12.5904655680574,1.92237131142328,0.201505034436202));
#10860=CARTESIAN_POINT('Ctrl Pts',(12.580927066184,1.91180972083614,0.403099401877819));
#10861=CARTESIAN_POINT('Ctrl Pts',(12.5713887230828,1.90124815518927,0.604693778165146));
#10862=CARTESIAN_POINT('Ctrl Pts',(12.6963322449987,1.94307475200582,-6.02899321996874E-5));
#10863=CARTESIAN_POINT('Ctrl Pts',(12.6866401583644,1.93251321719085,0.201534116525599));
#10864=CARTESIAN_POINT('Ctrl Pts',(12.6769482300299,1.921951707416,0.403128531931383));
#10865=CARTESIAN_POINT('Ctrl Pts',(12.6672564622458,1.91139022316341,0.604722956418908));
#10866=CARTESIAN_POINT('Ctrl Pts',(12.7926629650567,1.95339909479374,-3.05216148420481E-5));
#10867=CARTESIAN_POINT('Ctrl Pts',(12.7828174539371,1.94283764251631,0.201563933751552));
#10868=CARTESIAN_POINT('Ctrl Pts',(12.7729721028855,1.93227621586597,0.403158398304112));
#10869=CARTESIAN_POINT('Ctrl Pts',(12.7631269141765,1.92171481533599,0.604752872180064));
#10870=CARTESIAN_POINT('Ctrl Pts',(12.8889963716306,1.96391015057091,-1.66533453693773E-16));
#10871=CARTESIAN_POINT('Ctrl Pts',(12.878997439685,1.95334878321468,0.201594505478638));
#10872=CARTESIAN_POINT('Ctrl Pts',(12.8689986695886,1.94278744208894,0.403189020387166));
#10873=CARTESIAN_POINT('Ctrl Pts',(12.8590000636404,1.93222612769835,0.604783544866446));
#10874=CARTESIAN_POINT('',(12.8572578715866,1.93204080633595,0.60466226999893));
#10875=CARTESIAN_POINT('Ctrl Pts',(12.8889963716306,1.96391015057091,-3.88144377749811E-17));
#10876=CARTESIAN_POINT('Ctrl Pts',(12.8784169445746,1.95328733374019,0.201554108835021));
#10877=CARTESIAN_POINT('Ctrl Pts',(12.867837444884,1.94266422047353,0.403108198925375));
#10878=CARTESIAN_POINT('Ctrl Pts',(12.8572578715866,1.93204080633595,0.604662269998929));
#10879=CARTESIAN_POINT('Ctrl Pts',(12.8572578715866,1.93204080633595,0.60466226999893));
#10880=CARTESIAN_POINT('Ctrl Pts',(12.7715225733429,1.92264108900731,0.604675979983877));
#10881=CARTESIAN_POINT('Ctrl Pts',(12.6857696261193,1.91338852735451,0.604689390578107));
#10882=CARTESIAN_POINT('Ctrl Pts',(12.6000000000242,1.90428042250026,0.604702508168697));
#10883=CARTESIAN_POINT('Origin',(8.7,1.68851851851852,0.));
#10884=CARTESIAN_POINT('',(8.7,-1.5805153611151,0.605119933308333));
#10885=CARTESIAN_POINT('Ctrl Pts',(8.7,-1.5805153611151,0.605119933308333));
#10886=CARTESIAN_POINT('Ctrl Pts',(8.7,-1.58569938832865,0.504197823486131));
#10887=CARTESIAN_POINT('Ctrl Pts',(8.7,-1.59088373519313,0.403275164205241));
#10888=CARTESIAN_POINT('Ctrl Pts',(8.7,-1.60124586355191,0.201568897935389));
#10889=CARTESIAN_POINT('Ctrl Pts',(8.7,-1.60642370224807,0.10078416210737));
#10890=CARTESIAN_POINT('Ctrl Pts',(8.7,-1.61160179736194,0.));
#10891=CARTESIAN_POINT('',(8.7,-1.48045180431786,0.7));
#10892=CARTESIAN_POINT('Ctrl Pts',(8.70000000036779,-1.48045180452391,0.7));
#10893=CARTESIAN_POINT('Ctrl Pts',(8.70000000202598,-1.48836706478042,0.699999999180279));
#10894=CARTESIAN_POINT('Ctrl Pts',(8.70000127066624,-1.49622113223642,0.699007614827928));
#10895=CARTESIAN_POINT('Ctrl Pts',(8.70000237141531,-1.50387364922569,0.697121884028934));
#10896=CARTESIAN_POINT('Ctrl Pts',(8.70000291188189,-1.50763102664002,0.696195992283305));
#10897=CARTESIAN_POINT('Ctrl Pts',(8.70000341240591,-1.51133980954515,0.695053883793301));
#10898=CARTESIAN_POINT('Ctrl Pts',(8.70000377175886,-1.51498230649063,0.693702880475192));
#10899=CARTESIAN_POINT('Ctrl Pts',(8.70000450976793,-1.52246296255016,0.690928302676144));
#10900=CARTESIAN_POINT('Ctrl Pts',(8.70000452394134,-1.52958344744078,0.687306123577328));
#10901=CARTESIAN_POINT('Ctrl Pts',(8.70000379461986,-1.53619834892264,0.682919715776694));
#10902=CARTESIAN_POINT('Ctrl Pts',(8.70000333219987,-1.54039247012311,0.680138551763745));
#10903=CARTESIAN_POINT('Ctrl Pts',(8.70000258238552,-1.54438316197938,0.67704909562189));
#10904=CARTESIAN_POINT('Ctrl Pts',(8.70000192913237,-1.54812716280968,0.67366362845569));
#10905=CARTESIAN_POINT('Ctrl Pts',(8.70000138361353,-1.55125370412533,0.670836491537814));
#10906=CARTESIAN_POINT('Ctrl Pts',(8.70000090341281,-1.55418891097064,0.66782012731024));
#10907=CARTESIAN_POINT('Ctrl Pts',(8.7000009033621,-1.55691103280728,0.664625500020687));
#10908=CARTESIAN_POINT('Ctrl Pts',(8.7000009032669,-1.56202159382457,0.658627848677152));
#10909=CARTESIAN_POINT('Ctrl Pts',(8.70000241148087,-1.56638404855443,0.652003279246098));
#10910=CARTESIAN_POINT('Ctrl Pts',(8.70000292788623,-1.5699383402149,0.64491699469699));
#10911=CARTESIAN_POINT('Ctrl Pts',(8.70000298354275,-1.57032141040405,0.644153257609021));
#10912=CARTESIAN_POINT('Ctrl Pts',(8.70000303046442,-1.57069504840788,0.643384135640712));
#10913=CARTESIAN_POINT('Ctrl Pts',(8.70000306761332,-1.57105914547653,0.642609822781892));
#10914=CARTESIAN_POINT('Ctrl Pts',(8.70000341208914,-1.57443535963509,0.635429742901602));
#10915=CARTESIAN_POINT('Ctrl Pts',(8.70000263566904,-1.57695592401075,0.627888404173009));
#10916=CARTESIAN_POINT('Ctrl Pts',(8.70000151703179,-1.57856725066757,0.620153930269154));
#10917=CARTESIAN_POINT('Ctrl Pts',(8.70000080174396,-1.57959757782623,0.615208292159515));
#10918=CARTESIAN_POINT('Ctrl Pts',(8.7,-1.58025528705454,0.610183028431161));
#10919=CARTESIAN_POINT('Ctrl Pts',(8.7,-1.5805153611151,0.605119933308333));
#10920=CARTESIAN_POINT('',(8.7,1.48045180431904,0.7));
#10921=CARTESIAN_POINT('',(8.7,0.844259259259259,0.7));
#10922=CARTESIAN_POINT('',(8.7,1.5805153611151,0.605119933308333));
#10923=CARTESIAN_POINT('Ctrl Pts',(8.7,1.5805153611151,0.605119933308333));
#10924=CARTESIAN_POINT('Ctrl Pts',(8.7,1.58010890623597,0.61303275518587));
#10925=CARTESIAN_POINT('Ctrl Pts',(8.70000179355525,1.57873376841273,0.620855553142259));
#10926=CARTESIAN_POINT('Ctrl Pts',(8.7000025961206,1.5764741717406,0.62842799710221));
#10927=CARTESIAN_POINT('Ctrl Pts',(8.70000304562639,1.57520860278123,0.632669218617747));
#10928=CARTESIAN_POINT('Ctrl Pts',(8.70000324668712,1.57366457852079,0.636831947144834));
#10929=CARTESIAN_POINT('Ctrl Pts',(8.70000313318341,1.57185009366145,0.640886032861668));
#10930=CARTESIAN_POINT('Ctrl Pts',(8.70000293045856,1.56860930815545,0.648126888117959));
#10931=CARTESIAN_POINT('Ctrl Pts',(8.70000158438082,1.56454425420738,0.654942317779106));
#10932=CARTESIAN_POINT('Ctrl Pts',(8.70000106269264,1.55971945710293,0.661169479919421));
#10933=CARTESIAN_POINT('Ctrl Pts',(8.70000096439252,1.55881033523018,0.662342845179011));
#10934=CARTESIAN_POINT('Ctrl Pts',(8.70000090351839,1.55787410801649,0.663495254390581));
#10935=CARTESIAN_POINT('Ctrl Pts',(8.70000090409683,1.55691103285321,0.664625500020665));
#10936=CARTESIAN_POINT('Ctrl Pts',(8.70000090523835,1.55501044337284,0.666855993586132));
#10937=CARTESIAN_POINT('Ctrl Pts',(8.70000114361209,1.55300532702719,0.669000219206223));
#10938=CARTESIAN_POINT('Ctrl Pts',(8.70000146777886,1.55090303951829,0.671054438207787));
#10939=CARTESIAN_POINT('Ctrl Pts',(8.70000234447876,1.54521746205001,0.676610015749294));
#10940=CARTESIAN_POINT('Ctrl Pts',(8.70000370702799,1.53888821826629,0.681447385411957));
#10941=CARTESIAN_POINT('Ctrl Pts',(8.70000415375638,1.53207947242364,0.685512859850771));
#10942=CARTESIAN_POINT('Ctrl Pts',(8.70000443876751,1.52773551673798,0.688106618115728));
#10943=CARTESIAN_POINT('Ctrl Pts',(8.70000441165582,1.52319541573235,0.690385508075002));
#10944=CARTESIAN_POINT('Ctrl Pts',(8.70000407315693,1.51849599021366,0.692326230693156));
#10945=CARTESIAN_POINT('Ctrl Pts',(8.70000354533424,1.51116815716702,0.695352407250086));
#10946=CARTESIAN_POINT('Ctrl Pts',(8.70000225790696,1.50353761203248,0.697524030080351));
#10947=CARTESIAN_POINT('Ctrl Pts',(8.70000121423997,1.49575164755759,0.698771658000832));
#10948=CARTESIAN_POINT('Ctrl Pts',(8.70000053774506,1.49070486028667,0.699580358416591));
#10949=CARTESIAN_POINT('Ctrl Pts',(8.70000000144466,1.48559217323052,0.699999999467653));
#10950=CARTESIAN_POINT('Ctrl Pts',(8.70000000036779,1.48045180452391,0.7));
#10951=CARTESIAN_POINT('Ctrl Pts',(8.7,1.61160179736194,0.));
#10952=CARTESIAN_POINT('Ctrl Pts',(8.7,1.60642368739695,0.100784451162898));
#10953=CARTESIAN_POINT('Ctrl Pts',(8.7,1.60124583384883,0.201569476094892));
#10954=CARTESIAN_POINT('Ctrl Pts',(8.7,1.59088370548997,0.403275742430776));
#10955=CARTESIAN_POINT('Ctrl Pts',(8.7,1.58569937347746,0.504198112607714));
#10956=CARTESIAN_POINT('Ctrl Pts',(8.7,1.5805153611151,0.605119933308333));
#10957=CARTESIAN_POINT('Ctrl Pts',(8.7100201910492,-1.61222456240079,1.33887903992595E-6));
#10958=CARTESIAN_POINT('Ctrl Pts',(8.70667727354472,-1.60164608969543,0.201874135619687));
#10959=CARTESIAN_POINT('Ctrl Pts',(8.70333445073708,-1.59106762573893,0.40374693439627));
#10960=CARTESIAN_POINT('Ctrl Pts',(8.69999172399519,-1.58048917070122,0.605619735240497));
#10961=CARTESIAN_POINT('Ctrl Pts',(7.30266630830786,-1.52469223633113,-0.000186944012493601));
#10962=CARTESIAN_POINT('Ctrl Pts',(7.3015714609838,-1.51411327886182,0.201685539385837));
#10963=CARTESIAN_POINT('Ctrl Pts',(7.30047669312962,-1.50353432123569,0.403558023359813));
#10964=CARTESIAN_POINT('Ctrl Pts',(7.2993819983171,-1.49295537435081,0.605430507723141));
#10965=CARTESIAN_POINT('Ctrl Pts',(5.89591889571946,-1.46411055243784,-0.000276130330627546));
#10966=CARTESIAN_POINT('Ctrl Pts',(5.8970730573458,-1.45353136553189,0.201596203763285));
#10967=CARTESIAN_POINT('Ctrl Pts',(5.89822728315403,-1.44295217665945,0.403468537584815));
#10968=CARTESIAN_POINT('Ctrl Pts',(5.89938156763751,-1.43237299696387,0.60534087113472));
#10969=CARTESIAN_POINT('Ctrl Pts',(4.48978738186403,-1.41740792524342,-0.000330195618103912));
#10970=CARTESIAN_POINT('Ctrl Pts',(4.49319153668887,-1.4068286019831,0.201542048187911));
#10971=CARTESIAN_POINT('Ctrl Pts',(4.49659574248722,-1.39624928130228,0.403414291272231));
#10972=CARTESIAN_POINT('Ctrl Pts',(4.5,-1.3856699632509,0.605286533625018));
#10973=CARTESIAN_POINT('Ctrl Pts',(4.50000000014037,-1.38566996330298,0.605286533623957));
#10974=CARTESIAN_POINT('Ctrl Pts',(5.90109530155974,-1.43243455365708,0.605259331490037));
#10975=CARTESIAN_POINT('Ctrl Pts',(7.30150776148394,-1.49309969195427,0.605214402664297));
#10976=CARTESIAN_POINT('Ctrl Pts',(8.7,-1.5805153611151,0.605119933308333));
#10977=CARTESIAN_POINT('Ctrl Pts',(8.7062300060629,-1.48084102486261,0.7));
#10978=CARTESIAN_POINT('Ctrl Pts',(7.30535837857749,-1.39328148786737,0.7));
#10979=CARTESIAN_POINT('Ctrl Pts',(5.90286553803659,-1.3325543763676,0.7));
#10980=CARTESIAN_POINT('Ctrl Pts',(4.5,-1.28575421950843,0.7));
#10981=CARTESIAN_POINT('Ctrl Pts',(8.7044244076592,-1.50972892972339,0.7));
#10982=CARTESIAN_POINT('Ctrl Pts',(7.30392377861185,-1.42217417124324,0.699999322371676));
#10983=CARTESIAN_POINT('Ctrl Pts',(5.90170976758769,-1.36144968116949,0.700000194339816));
#10984=CARTESIAN_POINT('Ctrl Pts',(4.49903600403804,-1.314650633636,0.7));
#10985=CARTESIAN_POINT('Ctrl Pts',(8.70129509098077,-1.55979510296572,0.676577193851887));
#10986=CARTESIAN_POINT('Ctrl Pts',(7.30143307762773,-1.47225060169427,0.676608218952397));
#10987=CARTESIAN_POINT('Ctrl Pts',(5.89970879741633,-1.41153023905743,0.676622651488038));
#10988=CARTESIAN_POINT('Ctrl Pts',(4.49736521340071,-1.36473368385825,0.676631564755462));
#10989=CARTESIAN_POINT('Ctrl Pts',(8.70006933407556,-1.57940608001781,0.626799670546273));
#10990=CARTESIAN_POINT('Ctrl Pts',(7.3004573192207,-1.49190036240803,0.626879818917698));
#10991=CARTESIAN_POINT('Ctrl Pts',(5.89892183391985,-1.43119871194172,0.62691759730524));
#10992=CARTESIAN_POINT('Ctrl Pts',(4.49670869913724,-1.38441313147668,0.626940642142451));
#10993=CARTESIAN_POINT('Ctrl Pts',(8.7,-1.5805153611151,0.605119933308333));
#10994=CARTESIAN_POINT('Ctrl Pts',(7.30039998287682,-1.49303044794594,0.605214477495697));
#10995=CARTESIAN_POINT('Ctrl Pts',(5.89887670103551,-1.4323384618751,0.605259402637312));
#10996=CARTESIAN_POINT('Ctrl Pts',(4.49667047719213,-1.38555885946567,0.605286598232956));
#10997=CARTESIAN_POINT('Ctrl Pts',(8.70000000036771,-1.48045180452391,0.7));
#10998=CARTESIAN_POINT('Ctrl Pts',(7.30120024114866,-1.39310147361351,0.7));
#10999=CARTESIAN_POINT('Ctrl Pts',(5.90078591724148,-1.332484999384,0.7));
#11000=CARTESIAN_POINT('Ctrl Pts',(4.5,-1.28575421950843,0.7));
#11001=CARTESIAN_POINT('Origin',(6.87409734069396,-2.22251806091942E-16,
0.7));
#11002=CARTESIAN_POINT('Ctrl Pts',(4.5,1.28575421950843,0.7));
#11003=CARTESIAN_POINT('Ctrl Pts',(5.9007859172415,1.332484999384,0.7));
#11004=CARTESIAN_POINT('Ctrl Pts',(7.30120024114871,1.39310147361351,0.7));
#11005=CARTESIAN_POINT('Ctrl Pts',(8.70000000036779,1.48045180452391,0.7));
#11006=CARTESIAN_POINT('Ctrl Pts',(4.5,1.28575421950843,0.7));
#11007=CARTESIAN_POINT('Ctrl Pts',(5.90286553803659,1.3325543763676,0.7));
#11008=CARTESIAN_POINT('Ctrl Pts',(7.30535837857749,1.39328148786737,0.7));
#11009=CARTESIAN_POINT('Ctrl Pts',(8.7062300060629,1.48084102486261,0.7));
#11010=CARTESIAN_POINT('Ctrl Pts',(4.49903600403804,1.314650633636,0.7));
#11011=CARTESIAN_POINT('Ctrl Pts',(5.90170976758769,1.36144968116949,0.700000194339816));
#11012=CARTESIAN_POINT('Ctrl Pts',(7.30392377861185,1.42217417124324,0.699999322371676));
#11013=CARTESIAN_POINT('Ctrl Pts',(8.7044244076592,1.50972892972339,0.7));
#11014=CARTESIAN_POINT('Ctrl Pts',(4.49736521340071,1.36473368385825,0.676631564755462));
#11015=CARTESIAN_POINT('Ctrl Pts',(5.89970879741633,1.41153023905743,0.676622651488038));
#11016=CARTESIAN_POINT('Ctrl Pts',(7.30143307762774,1.47225060169427,0.676608218952397));
#11017=CARTESIAN_POINT('Ctrl Pts',(8.70129509098078,1.55979510296572,0.676577193851887));
#11018=CARTESIAN_POINT('Ctrl Pts',(4.49670869913724,1.38441313147668,0.626940642142451));
#11019=CARTESIAN_POINT('Ctrl Pts',(5.89892183391985,1.43119871194172,0.626917597305239));
#11020=CARTESIAN_POINT('Ctrl Pts',(7.3004573192207,1.49190036240803,0.626879818917698));
#11021=CARTESIAN_POINT('Ctrl Pts',(8.70006933407556,1.57940608001781,0.626799670546273));
#11022=CARTESIAN_POINT('Ctrl Pts',(4.49667047719213,1.38555885946567,0.605286598232956));
#11023=CARTESIAN_POINT('Ctrl Pts',(5.89887670103551,1.4323384618751,0.605259402637312));
#11024=CARTESIAN_POINT('Ctrl Pts',(7.30039998287682,1.49303044794594,0.605214477495697));
#11025=CARTESIAN_POINT('Ctrl Pts',(8.7,1.5805153611151,0.605119933308333));
#11026=CARTESIAN_POINT('Ctrl Pts',(8.7,1.5805153611151,0.605119933308333));
#11027=CARTESIAN_POINT('Ctrl Pts',(7.30150776148394,1.49309969195427,0.605214402664297));
#11028=CARTESIAN_POINT('Ctrl Pts',(5.90109530155974,1.43243455365708,0.605259331490037));
#11029=CARTESIAN_POINT('Ctrl Pts',(4.50000000014037,1.38566996330298,0.605286533623957));
#11030=CARTESIAN_POINT('Ctrl Pts',(4.48978738186405,1.41740792524342,-0.00033019561810394));
#11031=CARTESIAN_POINT('Ctrl Pts',(4.49319153668889,1.40682860198312,0.201542048187577));
#11032=CARTESIAN_POINT('Ctrl Pts',(4.49659574248723,1.39624928130232,0.403414291271564));
#11033=CARTESIAN_POINT('Ctrl Pts',(4.5,1.38566996325095,0.605286533624017));
#11034=CARTESIAN_POINT('Ctrl Pts',(5.89591889571947,1.46411055243784,-0.000276130330627574));
#11035=CARTESIAN_POINT('Ctrl Pts',(5.89707305734581,1.45353136553191,0.201596203762952));
#11036=CARTESIAN_POINT('Ctrl Pts',(5.89822728315404,1.44295217665948,0.403468537584147));
#11037=CARTESIAN_POINT('Ctrl Pts',(5.89938156763751,1.43237299696393,0.605340871133719));
#11038=CARTESIAN_POINT('Ctrl Pts',(7.30266630830786,1.52469223633113,-0.000186944012493549));
#11039=CARTESIAN_POINT('Ctrl Pts',(7.3015714609838,1.51411327886184,0.201685539385503));
#11040=CARTESIAN_POINT('Ctrl Pts',(7.30047669312963,1.50353432123572,0.403558023359145));
#11041=CARTESIAN_POINT('Ctrl Pts',(7.29938199831711,1.49295537435086,0.60543050772214));
#11042=CARTESIAN_POINT('Ctrl Pts',(8.7100201910492,1.61222456240079,1.33887903989646E-6));
#11043=CARTESIAN_POINT('Ctrl Pts',(8.70667727354472,1.60164608969545,0.201874135619353));
#11044=CARTESIAN_POINT('Ctrl Pts',(8.7033344507371,1.59106762573896,0.403746934395602));
#11045=CARTESIAN_POINT('Ctrl Pts',(8.6999917239952,1.58048917070127,0.605619735239495));
#11046=CARTESIAN_POINT('Origin',(4.3,1.48481481481482,0.));
#11047=CARTESIAN_POINT('',(4.3,-1.37908752581626,0.605290299758539));
#11048=CARTESIAN_POINT('Ctrl Pts',(4.3,-1.37908752581626,0.605290299758539));
#11049=CARTESIAN_POINT('Ctrl Pts',(4.3,-1.38444464017247,0.504222347694443));
#11050=CARTESIAN_POINT('Ctrl Pts',(4.3,-1.38980163214303,0.403154389143214));
#11051=CARTESIAN_POINT('Ctrl Pts',(4.3,-1.40049562949383,0.201390955816302));
#11052=CARTESIAN_POINT('Ctrl Pts',(4.3,-1.40583263576898,0.100695481088992));
#11053=CARTESIAN_POINT('Ctrl Pts',(4.3,-1.41116952203211,0.));
#11054=CARTESIAN_POINT('Ctrl Pts',(4.30000000005992,-1.27917501058303,0.7));
#11055=CARTESIAN_POINT('Ctrl Pts',(4.30000000048661,-1.28708628524264,0.699999999884766));
#11056=CARTESIAN_POINT('Ctrl Pts',(4.30000064978116,-1.29493415608545,0.69900616264686));
#11057=CARTESIAN_POINT('Ctrl Pts',(4.30000121018478,-1.30257825621016,0.697119208693397));
#11058=CARTESIAN_POINT('Ctrl Pts',(4.30000152558655,-1.30688044586137,0.696057208766858));
#11059=CARTESIAN_POINT('Ctrl Pts',(4.30000181105247,-1.31111814675806,0.694711271736901));
#11060=CARTESIAN_POINT('Ctrl Pts',(4.30000199036827,-1.31526464671957,0.693092387263961));
#11061=CARTESIAN_POINT('Ctrl Pts',(4.30000231141323,-1.32268849323592,0.690193954859197));
#11062=CARTESIAN_POINT('Ctrl Pts',(4.30000222777046,-1.32973966400828,0.686455190804221));
#11063=CARTESIAN_POINT('Ctrl Pts',(4.30000179417102,-1.33627196700415,0.681957645816867));
#11064=CARTESIAN_POINT('Ctrl Pts',(4.30000155535849,-1.33986974800182,0.679480543652151));
#11065=CARTESIAN_POINT('Ctrl Pts',(4.30000121902461,-1.34330986828215,0.67677238407294));
#11066=CARTESIAN_POINT('Ctrl Pts',(4.30000092191081,-1.34656397897095,0.673841242448196));
#11067=CARTESIAN_POINT('Ctrl Pts',(4.30000063243573,-1.34973442737118,0.670985459666446));
#11068=CARTESIAN_POINT('Ctrl Pts',(4.30000037658882,-1.35270906921767,0.667935271966333));
#11069=CARTESIAN_POINT('Ctrl Pts',(4.30000037869864,-1.35546536049262,0.66470214425512));
#11070=CARTESIAN_POINT('Ctrl Pts',(4.30000038260995,-1.36057515211559,0.658708362304413));
#11071=CARTESIAN_POINT('Ctrl Pts',(4.30000117797282,-1.36493744806469,0.652087250959406));
#11072=CARTESIAN_POINT('Ctrl Pts',(4.30000145944905,-1.36849285270534,0.645004510397983));
#11073=CARTESIAN_POINT('Ctrl Pts',(4.30000148826005,-1.36885677248754,0.644279543857467));
#11074=CARTESIAN_POINT('Ctrl Pts',(4.30000151299237,-1.36921219826683,0.643549721050429));
#11075=CARTESIAN_POINT('Ctrl Pts',(4.30000153317099,-1.36955903781249,0.642815208524159));
#11076=CARTESIAN_POINT('Ctrl Pts',(4.30000173031152,-1.37294758118467,0.635639188419686));
#11077=CARTESIAN_POINT('Ctrl Pts',(4.30000134819424,-1.37548140076902,0.628100134775109));
#11078=CARTESIAN_POINT('Ctrl Pts',(4.30000077902196,-1.37710733725971,0.620366659714886));
#11079=CARTESIAN_POINT('Ctrl Pts',(4.30000041405338,-1.37814993145247,0.615407747584041));
#11080=CARTESIAN_POINT('Ctrl Pts',(4.3,-1.37881837002099,0.610368224776708));
#11081=CARTESIAN_POINT('Ctrl Pts',(4.3,-1.37908752581626,0.605290299758539));
#11082=CARTESIAN_POINT('',(4.3,1.37908752581626,0.605290299758539));
#11083=CARTESIAN_POINT('Ctrl Pts',(4.3,1.37908752581626,0.605290299758539));
#11084=CARTESIAN_POINT('Ctrl Pts',(4.3,1.37866806817032,0.613203837240499));
#11085=CARTESIAN_POINT('Ctrl Pts',(4.30000092021544,1.37728139671899,0.621026590428679));
#11086=CARTESIAN_POINT('Ctrl Pts',(4.30000132151137,1.37501133257008,0.628597948954885));
#11087=CARTESIAN_POINT('Ctrl Pts',(4.30000154544343,1.37374458621782,0.632822935636113));
#11088=CARTESIAN_POINT('Ctrl Pts',(4.30000164013187,1.37220176226583,0.636969676056352));
#11089=CARTESIAN_POINT('Ctrl Pts',(4.30000157305315,1.37039070587839,0.641008268098125));
#11090=CARTESIAN_POINT('Ctrl Pts',(4.30000145288191,1.36714620633991,0.648243387946652));
#11091=CARTESIAN_POINT('Ctrl Pts',(4.30000073948134,1.36307905360626,0.655053358422861));
#11092=CARTESIAN_POINT('Ctrl Pts',(4.3000004635866,1.35825284513469,0.661274801567968));
#11093=CARTESIAN_POINT('Ctrl Pts',(4.30000041199046,1.35735027731582,0.662438297592388));
#11094=CARTESIAN_POINT('Ctrl Pts',(4.30000037986005,1.35642103364291,0.663581140343808));
#11095=CARTESIAN_POINT('Ctrl Pts',(4.30000037943224,1.35546536051643,0.664702144255114));
#11096=CARTESIAN_POINT('Ctrl Pts',(4.300000378582,1.3535659898678,0.666930104702213));
#11097=CARTESIAN_POINT('Ctrl Pts',(4.3000005018795,1.35156225525783,0.669071850305581));
#11098=CARTESIAN_POINT('Ctrl Pts',(4.30000067038034,1.34946148384904,0.671123623013939));
#11099=CARTESIAN_POINT('Ctrl Pts',(4.30000112630012,1.34377733881547,0.676675190215126));
#11100=CARTESIAN_POINT('Ctrl Pts',(4.30000183907902,1.33744971106208,0.68150833207295));
#11101=CARTESIAN_POINT('Ctrl Pts',(4.30000208123143,1.33064243458576,0.685568782013219));
#11102=CARTESIAN_POINT('Ctrl Pts',(4.30000223513396,1.3263159977886,0.688149444058562));
#11103=CARTESIAN_POINT('Ctrl Pts',(4.3000022300233,1.32179485563522,0.690417305529342));
#11104=CARTESIAN_POINT('Ctrl Pts',(4.30000206344016,1.31711540146937,0.692349146556373));
#11105=CARTESIAN_POINT('Ctrl Pts',(4.3000018029167,1.30979708846622,0.695370400063095));
#11106=CARTESIAN_POINT('Ctrl Pts',(4.30000114702936,1.30217656646843,0.69753735975804));
#11107=CARTESIAN_POINT('Ctrl Pts',(4.3000006156201,1.29440092269557,0.69878042986007));
#11108=CARTESIAN_POINT('Ctrl Pts',(4.30000027236218,1.28937833178082,0.699583377215073));
#11109=CARTESIAN_POINT('Ctrl Pts',(4.30000000033581,1.28429042584107,0.69999999992549));
#11110=CARTESIAN_POINT('Ctrl Pts',(4.30000000005992,1.27917501058303,0.7));
#11111=CARTESIAN_POINT('Ctrl Pts',(4.3,1.41116952203211,0.));
#11112=CARTESIAN_POINT('Ctrl Pts',(4.3,1.40583262613343,0.100695662891028));
#11113=CARTESIAN_POINT('Ctrl Pts',(4.3,1.40049561022223,0.201391319421434));
#11114=CARTESIAN_POINT('Ctrl Pts',(4.3,1.38980161287056,0.403154752748307));
#11115=CARTESIAN_POINT('Ctrl Pts',(4.3,1.38444463053604,0.504222529496425));
#11116=CARTESIAN_POINT('Ctrl Pts',(4.3,1.37908752581626,0.605290299758539));
#11117=CARTESIAN_POINT('Ctrl Pts',(4.3,-1.41116952203217,-1.08233907947231E-12));
#11118=CARTESIAN_POINT('Ctrl Pts',(4.30370667985561,-1.40059355144761,0.201807922462111));
#11119=CARTESIAN_POINT('Ctrl Pts',(4.30741340932898,-1.39001758331341,0.403615844144917));
#11120=CARTESIAN_POINT('Ctrl Pts',(4.31112018914117,-1.37944161767694,0.605423765036612));
#11121=CARTESIAN_POINT('Ctrl Pts',(3.22410085073145,-1.37636920007795,-3.90459529712038E-5));
#11122=CARTESIAN_POINT('Ctrl Pts',(3.2295286994181,-1.36579313421488,0.201768811380596));
#11123=CARTESIAN_POINT('Ctrl Pts',(3.23495659078338,-1.35521706809947,0.403576667516588));
#11124=CARTESIAN_POINT('Ctrl Pts',(3.24038452463065,-1.34464100578453,0.605384522622892));
#11125=CARTESIAN_POINT('Ctrl Pts',(2.14856196511704,-1.34935185539723,-5.92140864038068E-5));
#11126=CARTESIAN_POINT('Ctrl Pts',(2.15571155670467,-1.33877574824886,0.201748609775608));
#11127=CARTESIAN_POINT('Ctrl Pts',(2.16286118630165,-1.32819964054015,0.403556432267456));
#11128=CARTESIAN_POINT('Ctrl Pts',(2.17001085376486,-1.31762353633116,0.605364253566666));
#11129=CARTESIAN_POINT('Ctrl Pts',(1.073384157387,-1.32427529283232,-8.86713468529234E-5));
#11130=CARTESIAN_POINT('Ctrl Pts',(1.08225606990756,-1.31369916974321,0.201719104822629));
#11131=CARTESIAN_POINT('Ctrl Pts',(1.09112801825726,-1.30312304798914,0.403526879488275));
#11132=CARTESIAN_POINT('Ctrl Pts',(1.10000000295732,-1.29254692759565,0.605334652628532));
#11133=CARTESIAN_POINT('Ctrl Pts',(1.10000000298281,-1.29254692760111,0.605334652628557));
#11134=CARTESIAN_POINT('Ctrl Pts',(2.16694388170712,-1.31755402957363,0.605319894542965));
#11135=CARTESIAN_POINT('Ctrl Pts',(3.23367147240841,-1.34448060345116,0.605309774863278));
#11136=CARTESIAN_POINT('Ctrl Pts',(4.3,-1.37908752581626,0.605290299758539));
#11137=CARTESIAN_POINT('Ctrl Pts',(4.30323908112369,-1.2792801058419,0.7));
#11138=CARTESIAN_POINT('Ctrl Pts',(3.23565147654712,-1.24463335454069,0.7));
#11139=CARTESIAN_POINT('Ctrl Pts',(2.1678436779024,-1.21768649131741,0.7));
#11140=CARTESIAN_POINT('Ctrl Pts',(1.09999999999999,-1.19266190204553,0.7));
#11141=CARTESIAN_POINT('Ctrl Pts',(4.30230129178181,-1.30817667592415,0.7));
#11142=CARTESIAN_POINT('Ctrl Pts',(3.23485320804887,-1.27353066282864,0.699999860738333));
#11143=CARTESIAN_POINT('Ctrl Pts',(2.16713169816659,-1.24658393122273,0.700000105496227));
#11144=CARTESIAN_POINT('Ctrl Pts',(1.0993228455422,-1.22155728565617,0.7));
#11145=CARTESIAN_POINT('Ctrl Pts',(4.30067574076257,-1.35826558912881,0.676637683834297));
#11146=CARTESIAN_POINT('Ctrl Pts',(3.23346787205668,-1.32362126434549,0.676644071225102));
#11147=CARTESIAN_POINT('Ctrl Pts',(2.16589795861771,-1.29667457247055,0.676647306834711));
#11148=CARTESIAN_POINT('Ctrl Pts',(1.09814906228501,-1.27164470234869,0.676652147774997));
#11149=CARTESIAN_POINT('Ctrl Pts',(4.30003720890047,-1.37794098943329,0.626943772371838));
#11150=CARTESIAN_POINT('Ctrl Pts',(3.23292426239396,-1.34330449078822,0.626960286972675));
#11151=CARTESIAN_POINT('Ctrl Pts',(2.16541285690349,-1.31636171257899,0.6269687859393));
#11152=CARTESIAN_POINT('Ctrl Pts',(1.09768760301306,-1.29133598921902,0.626981304916489));
#11153=CARTESIAN_POINT('Ctrl Pts',(4.3,-1.37908752581626,0.605290299758539));
#11154=CARTESIAN_POINT('Ctrl Pts',(3.23289209128077,-1.34445530919946,0.605309789097661));
#11155=CARTESIAN_POINT('Ctrl Pts',(2.16538453588699,-1.31751467232976,0.605319909330946));
#11156=CARTESIAN_POINT('Ctrl Pts',(1.09766050997011,-1.29249209748956,0.605334684996117));
#11157=CARTESIAN_POINT('Ctrl Pts',(1.09999999999999,1.19266190204553,0.7));
#11158=CARTESIAN_POINT('Ctrl Pts',(2.1678436779024,1.21768649131741,0.7));
#11159=CARTESIAN_POINT('Ctrl Pts',(3.23565147654712,1.24463335454069,0.7));
#11160=CARTESIAN_POINT('Ctrl Pts',(4.30323908112369,1.2792801058419,0.7));
#11161=CARTESIAN_POINT('Ctrl Pts',(1.0993228455422,1.22155728565617,0.7));
#11162=CARTESIAN_POINT('Ctrl Pts',(2.16713169816659,1.24658393122273,0.700000105496227));
#11163=CARTESIAN_POINT('Ctrl Pts',(3.23485320804887,1.27353066282864,0.699999860738333));
#11164=CARTESIAN_POINT('Ctrl Pts',(4.30230129178181,1.30817667592415,0.7));
#11165=CARTESIAN_POINT('Ctrl Pts',(1.09814906228501,1.27164470234869,0.676652147774997));
#11166=CARTESIAN_POINT('Ctrl Pts',(2.16589795861771,1.29667457247055,0.676647306834711));
#11167=CARTESIAN_POINT('Ctrl Pts',(3.23346787205668,1.32362126434549,0.676644071225102));
#11168=CARTESIAN_POINT('Ctrl Pts',(4.30067574076257,1.35826558912881,0.676637683834297));
#11169=CARTESIAN_POINT('Ctrl Pts',(1.09768760301306,1.29133598921902,0.626981304916489));
#11170=CARTESIAN_POINT('Ctrl Pts',(2.16541285690349,1.31636171257899,0.6269687859393));
#11171=CARTESIAN_POINT('Ctrl Pts',(3.23292426239396,1.34330449078822,0.626960286972675));
#11172=CARTESIAN_POINT('Ctrl Pts',(4.30003720890047,1.37794098943329,0.626943772371838));
#11173=CARTESIAN_POINT('Ctrl Pts',(1.09766050997011,1.29249209748956,0.605334684996117));
#11174=CARTESIAN_POINT('Ctrl Pts',(2.16538453588699,1.31751467232976,0.605319909330946));
#11175=CARTESIAN_POINT('Ctrl Pts',(3.23289209128077,1.34445530919946,0.605309789097661));
#11176=CARTESIAN_POINT('Ctrl Pts',(4.3,1.37908752581626,0.605290299758539));
#11177=CARTESIAN_POINT('Ctrl Pts',(4.3,1.37908752581626,0.605290299758539));
#11178=CARTESIAN_POINT('Ctrl Pts',(3.23367147240841,1.34448060345116,0.605309774863278));
#11179=CARTESIAN_POINT('Ctrl Pts',(2.16694388170711,1.31755402957363,0.605319894542965));
#11180=CARTESIAN_POINT('Ctrl Pts',(1.10000000298281,1.29254692760111,0.605334652628557));
#11181=CARTESIAN_POINT('Ctrl Pts',(1.07338415738705,1.32427529283227,-8.86713457716078E-5));
#11182=CARTESIAN_POINT('Ctrl Pts',(1.08225606990759,1.31369916974318,0.201719104823349));
#11183=CARTESIAN_POINT('Ctrl Pts',(1.09112801825728,1.30312304798912,0.403526879488635));
#11184=CARTESIAN_POINT('Ctrl Pts',(1.10000000295732,1.29254692759565,0.605334652628532));
#11185=CARTESIAN_POINT('Ctrl Pts',(2.14856196511707,1.34935185539717,-5.92140853224782E-5));
#11186=CARTESIAN_POINT('Ctrl Pts',(2.15571155670469,1.33877574824882,0.201748609776328));
#11187=CARTESIAN_POINT('Ctrl Pts',(2.16286118630166,1.32819964054013,0.403556432267816));
#11188=CARTESIAN_POINT('Ctrl Pts',(2.17001085376486,1.31762353633116,0.605364253566666));
#11189=CARTESIAN_POINT('Ctrl Pts',(3.22410085073147,1.37636920007789,-3.90459518899617E-5));
#11190=CARTESIAN_POINT('Ctrl Pts',(3.22952869941811,1.36579313421484,0.201768811381317));
#11191=CARTESIAN_POINT('Ctrl Pts',(3.23495659078338,1.35521706809945,0.403576667516948));
#11192=CARTESIAN_POINT('Ctrl Pts',(3.24038452463064,1.34464100578453,0.605384522622892));
#11193=CARTESIAN_POINT('Ctrl Pts',(4.3,1.41116952203211,-1.07899800205757E-15));
#11194=CARTESIAN_POINT('Ctrl Pts',(4.3037066798556,1.40059355144758,0.201807922462832));
#11195=CARTESIAN_POINT('Ctrl Pts',(4.30741340932897,1.39001758331339,0.403615844145277));
#11196=CARTESIAN_POINT('Ctrl Pts',(4.31112018914115,1.37944161767694,0.605423765036611));
#11197=CARTESIAN_POINT('Origin',(0.9,1.39290118819044,0.));
#11198=CARTESIAN_POINT('',(0.900000001878204,-1.28788040994396,0.605337476551879));
#11199=CARTESIAN_POINT('Ctrl Pts',(0.900000001878204,-1.28788040994396,
0.605337476551879));
#11200=CARTESIAN_POINT('Ctrl Pts',(0.900000001878204,-1.29328625806092,
0.504228160928694));
#11201=CARTESIAN_POINT('Ctrl Pts',(0.899999999999999,-1.29869191435855,
0.403118132397745));
#11202=CARTESIAN_POINT('Ctrl Pts',(0.899999999999999,-1.30947917558554,
0.201339438823693));
#11203=CARTESIAN_POINT('Ctrl Pts',(0.9,-1.31486085669789,0.100669384150719));
#11204=CARTESIAN_POINT('Ctrl Pts',(0.9,-1.32024227787037,0.));
#11205=CARTESIAN_POINT('',(0.9,-1.18799600975353,0.7));
#11206=CARTESIAN_POINT('Ctrl Pts',(0.900000000000324,-1.18799600975363,
0.7));
#11207=CARTESIAN_POINT('Ctrl Pts',(0.900000000063601,-1.19590581948314,
0.699999999935493));
#11208=CARTESIAN_POINT('Ctrl Pts',(0.900000451671414,-1.20375274583281,
0.699006541951706));
#11209=CARTESIAN_POINT('Ctrl Pts',(0.900000834722547,-1.21139610511184,
0.697120084132161));
#11210=CARTESIAN_POINT('Ctrl Pts',(0.900001049758257,-1.21568690349652,
0.696061072005504));
#11211=CARTESIAN_POINT('Ctrl Pts',(0.900001241882928,-1.21991360580594,
0.694719604949841));
#11212=CARTESIAN_POINT('Ctrl Pts',(0.900001357948449,-1.22404965357203,
0.693106547509926));
#11213=CARTESIAN_POINT('Ctrl Pts',(0.900001566283472,-1.23147376710855,
0.690211145364658));
#11214=CARTESIAN_POINT('Ctrl Pts',(0.900001483882417,-1.23852542365708,
0.686475281350474));
#11215=CARTESIAN_POINT('Ctrl Pts',(0.90000115772027,-1.24505817055452,0.681980323292531));
#11216=CARTESIAN_POINT('Ctrl Pts',(0.90000097852015,-1.2486473946309,0.67951070187031));
#11217=CARTESIAN_POINT('Ctrl Pts',(0.900000731874511,-1.25207971535834,
0.676811055842604));
#11218=CARTESIAN_POINT('Ctrl Pts',(0.90000051586667,-1.25532695882913,0.673889369778116));
#11219=CARTESIAN_POINT('Ctrl Pts',(0.900000304282776,-1.25850769714062,
0.671027521295527));
#11220=CARTESIAN_POINT('Ctrl Pts',(0.900000119565725,-1.26149151526032,
0.667969976014938));
#11221=CARTESIAN_POINT('Ctrl Pts',(0.900000124706954,-1.26425564062679,
0.664728268702146));
#11222=CARTESIAN_POINT('Ctrl Pts',(0.900000134210909,-1.26936533657602,
0.658735726205464));
#11223=CARTESIAN_POINT('Ctrl Pts',(0.900000724431276,-1.2737272220214,0.652115259198653));
#11224=CARTESIAN_POINT('Ctrl Pts',(0.900000949945503,-1.27728244659665,
0.645033014705304));
#11225=CARTESIAN_POINT('Ctrl Pts',(0.900000972753073,-1.27764200720725,
0.644316745985709));
#11226=CARTESIAN_POINT('Ctrl Pts',(0.900000992743332,-1.27799327761064,
0.64359573459864));
#11227=CARTESIAN_POINT('Ctrl Pts',(0.900001009576454,-1.27833616945273,
0.642870141642621));
#11228=CARTESIAN_POINT('Ctrl Pts',(0.900001176059944,-1.28172744954266,
0.635693858502874));
#11229=CARTESIAN_POINT('Ctrl Pts',(0.900000930108723,-1.28426399347052,
0.628153947608977));
#11230=CARTESIAN_POINT('Ctrl Pts',(0.900000539908504,-1.2858931319598,0.620419547606466));
#11231=CARTESIAN_POINT('Ctrl Pts',(0.900000289636433,-1.28693805157347,
0.615458750034127));
#11232=CARTESIAN_POINT('Ctrl Pts',(0.900000000000001,-1.28760881677759,
0.610417269724172));
#11233=CARTESIAN_POINT('Ctrl Pts',(0.900000000000001,-1.28788040985668,
0.605337476551933));
#11234=CARTESIAN_POINT('',(0.9,1.18799600975353,0.7));
#11235=CARTESIAN_POINT('',(0.9,0.696450594095222,0.7));
#11236=CARTESIAN_POINT('',(0.900000001878204,1.28788040994396,0.605337476551879));
#11237=CARTESIAN_POINT('Ctrl Pts',(0.900000000000001,1.28788040985668,0.605337476551933));
#11238=CARTESIAN_POINT('Ctrl Pts',(0.900000000000001,1.28745726486871,0.613251849878237));
#11239=CARTESIAN_POINT('Ctrl Pts',(0.900000641820462,1.28606767879774,0.621075732439556));
#11240=CARTESIAN_POINT('Ctrl Pts',(0.900000906166769,1.28379497466322,0.628648019961568));
#11241=CARTESIAN_POINT('Ctrl Pts',(0.900001053446495,1.2825287445946,0.632866896498568));
#11242=CARTESIAN_POINT('Ctrl Pts',(0.900001106693909,1.28098738700664,0.637007708770872));
#11243=CARTESIAN_POINT('Ctrl Pts',(0.900001044867119,1.27917862712792,0.641040603354488));
#11244=CARTESIAN_POINT('Ctrl Pts',(0.900000933962191,1.27593407274945,0.64827481168313));
#11245=CARTESIAN_POINT('Ctrl Pts',(0.900000399592996,1.27186725264719,0.655083885116145));
#11246=CARTESIAN_POINT('Ctrl Pts',(0.900000190596867,1.2670411556595,0.661303993035384));
#11247=CARTESIAN_POINT('Ctrl Pts',(0.900000151538061,1.26613921747962,0.662466454716044));
#11248=CARTESIAN_POINT('Ctrl Pts',(0.900000126821978,1.26521063179286,0.663608275427336));
#11249=CARTESIAN_POINT('Ctrl Pts',(0.900000125264574,1.26425564063975,0.664728268702142));
#11250=CARTESIAN_POINT('Ctrl Pts',(0.90000012217056,1.26235840892454,0.66695330163032));
#11251=CARTESIAN_POINT('Ctrl Pts',(0.900000209712012,1.26035699384613,0.66909223571964));
#11252=CARTESIAN_POINT('Ctrl Pts',(0.900000331194293,1.2582587086698,0.671141334714948));
#11253=CARTESIAN_POINT('Ctrl Pts',(0.900000660246931,1.25257519443757,0.676691620936499));
#11254=CARTESIAN_POINT('Ctrl Pts',(0.900001184896248,1.24624785575673,0.681523125886843));
#11255=CARTESIAN_POINT('Ctrl Pts',(0.900001377531805,1.23944073409582,0.685581770965975));
#11256=CARTESIAN_POINT('Ctrl Pts',(0.900001499905572,1.2351164383281,0.68816006802201));
#11257=CARTESIAN_POINT('Ctrl Pts',(0.900001510509735,1.23059756718463,0.690425789971136));
#11258=CARTESIAN_POINT('Ctrl Pts',(0.900001405318139,1.22592052877826,0.692355791713551));
#11259=CARTESIAN_POINT('Ctrl Pts',(0.900001240727996,1.21860250674997,0.695375607682216));
#11260=CARTESIAN_POINT('Ctrl Pts',(0.900000792095824,1.21098234272326,0.697541065921879));
#11261=CARTESIAN_POINT('Ctrl Pts',(0.900000425437202,1.20320741268883,0.698782789564668));
#11262=CARTESIAN_POINT('Ctrl Pts',(0.900000188792485,1.19818940410026,0.699584208982791));
#11263=CARTESIAN_POINT('Ctrl Pts',(0.900000000041206,1.19310633605572,0.699999999958324));
#11264=CARTESIAN_POINT('Ctrl Pts',(0.900000000000325,1.18799600975363,0.7));
#11265=CARTESIAN_POINT('Ctrl Pts',(0.9,1.32024227787037,0.));
#11266=CARTESIAN_POINT('Ctrl Pts',(0.9,1.31486080448354,0.100670360916234));
#11267=CARTESIAN_POINT('Ctrl Pts',(0.9,1.30947907114291,0.201341392534));
#11268=CARTESIAN_POINT('Ctrl Pts',(0.9,1.2986918099064,0.403120086121531));
#11269=CARTESIAN_POINT('Ctrl Pts',(0.900000001878204,1.29328620583358,0.504229137772713));
#11270=CARTESIAN_POINT('Ctrl Pts',(0.900000001878204,1.28788040994396,0.605337476551879));
#11271=CARTESIAN_POINT('Ctrl Pts',(0.899999999999997,-1.32024227787137,
-1.86669707469278E-11));
#11272=CARTESIAN_POINT('Ctrl Pts',(0.909148787559422,-1.30966717532842,
0.201788252636133));
#11273=CARTESIAN_POINT('Ctrl Pts',(0.91829761066914,-1.29909207410335,0.403576503749508));
#11274=CARTESIAN_POINT('Ctrl Pts',(0.92744646984625,-1.28851697422138,0.605364753299354));
#11275=CARTESIAN_POINT('Ctrl Pts',(0.699273108318574,-1.31559634352334,
-5.7001548815619E-6));
#11276=CARTESIAN_POINT('Ctrl Pts',(0.708743431409066,-1.30502123870946,
0.20178254329682));
#11277=CARTESIAN_POINT('Ctrl Pts',(0.718213789763005,-1.2944461351935,0.403570785162392));
#11278=CARTESIAN_POINT('Ctrl Pts',(0.727684183892774,-1.28387103300525,
0.605359025419352));
#11279=CARTESIAN_POINT('Ctrl Pts',(0.498558799217305,-1.31100715552056,
-1.1774619888836E-5));
#11280=CARTESIAN_POINT('Ctrl Pts',(0.508350677965937,-1.30043204942944,
0.201776459055217));
#11281=CARTESIAN_POINT('Ctrl Pts',(0.518142591787393,-1.28985694462582,
0.403564691096996));
#11282=CARTESIAN_POINT('Ctrl Pts',(0.527934541191295,-1.27928184113929,
0.60535292148228));
#11283=CARTESIAN_POINT('Ctrl Pts',(0.29785707328833,-1.3064367443434,-1.84041486642056E-5));
#11284=CARTESIAN_POINT('Ctrl Pts',(0.307970527825607,-1.29586163794,0.20176981888596));
#11285=CARTESIAN_POINT('Ctrl Pts',(0.318084017341356,-1.28528653282298,
0.403558040236175));
#11286=CARTESIAN_POINT('Ctrl Pts',(0.328197542344371,-1.27471142901691,
0.605346259877786));
#11287=CARTESIAN_POINT('',(0.32957180616905,-1.2747428754212,0.605346305703265));
#11288=CARTESIAN_POINT('Ctrl Pts',(0.297857995688647,-1.306435779838,1.57426155444895E-16));
#11289=CARTESIAN_POINT('Ctrl Pts',(0.308429283449307,-1.29587142805659,
0.201782098465301));
#11290=CARTESIAN_POINT('Ctrl Pts',(0.319000553694994,-1.28530712634462,
0.403564200350135));
#11291=CARTESIAN_POINT('Ctrl Pts',(0.329571806169048,-1.2747428754212,0.605346305703266));
#11292=CARTESIAN_POINT('Ctrl Pts',(0.32957180616905,-1.2747428754212,0.605346305703265));
#11293=CARTESIAN_POINT('Ctrl Pts',(0.519721397561595,-1.27909449722757,
0.60534313598158));
#11294=CARTESIAN_POINT('Ctrl Pts',(0.709864288600121,-1.28346276435313,
0.605340219076093));
#11295=CARTESIAN_POINT('Ctrl Pts',(0.900000001879218,-1.28788040990034,
0.605337476551906));
#11296=CARTESIAN_POINT('Ctrl Pts',(0.90231940407953,-1.18804989493878,0.7));
#11297=CARTESIAN_POINT('Ctrl Pts',(0.712166351817731,-1.18363199317816,
0.7));
#11298=CARTESIAN_POINT('Ctrl Pts',(0.522011847238247,-1.17926361631973,
0.7));
#11299=CARTESIAN_POINT('Ctrl Pts',(0.331856371369203,-1.17491202960101,
0.7));
#11300=CARTESIAN_POINT('Ctrl Pts',(0.901648075315333,-1.21694488185794,
0.7));
#11301=CARTESIAN_POINT('Ctrl Pts',(0.711500071980331,-1.21252656425213,
0.69999998041973));
#11302=CARTESIAN_POINT('Ctrl Pts',(0.521348914609444,-1.20815772874132,
0.700000022626678));
#11303=CARTESIAN_POINT('Ctrl Pts',(0.331195161244126,-1.20380556524924,
0.7));
#11304=CARTESIAN_POINT('Ctrl Pts',(0.900484091294294,-1.26704448261357,
0.676664431332699));
#11305=CARTESIAN_POINT('Ctrl Pts',(0.710344780071471,-1.26262550764723,
0.676665329845182));
#11306=CARTESIAN_POINT('Ctrl Pts',(0.520199507967113,-1.25825584722226,
0.676666267597974));
#11307=CARTESIAN_POINT('Ctrl Pts',(0.3300487189482,-1.25390275839508,0.676667306001616));
#11308=CARTESIAN_POINT('Ctrl Pts',(0.90002687589075,-1.28672371253673,0.626983665342106));
#11309=CARTESIAN_POINT('Ctrl Pts',(0.709890987426059,-1.28230548388611,
0.626985988983916));
#11310=CARTESIAN_POINT('Ctrl Pts',(0.519747959090447,-1.27793661492756,
0.626988445273931));
#11311=CARTESIAN_POINT('Ctrl Pts',(0.329598318905021,-1.27358432286302,
0.626991130804315));
#11312=CARTESIAN_POINT('Ctrl Pts',(0.900000001879218,-1.28788040990034,
0.605337476551906));
#11313=CARTESIAN_POINT('Ctrl Pts',(0.709864288600121,-1.28346276435313,
0.605340219076093));
#11314=CARTESIAN_POINT('Ctrl Pts',(0.519721397561595,-1.27909449722757,
0.60534313598158));
#11315=CARTESIAN_POINT('Ctrl Pts',(0.32957180616905,-1.2747428754212,0.605346305703265));
#11316=CARTESIAN_POINT('',(0.331856371369201,-1.17491202962433,0.7));
#11317=CARTESIAN_POINT('Origin',(0.331856371539144,-1.1749120296049,0.6));
#11318=CARTESIAN_POINT('Ctrl Pts',(0.900000000000328,-1.18799600975363,
0.7));
#11319=CARTESIAN_POINT('Ctrl Pts',(0.71062007065371,-1.18359647108512,0.7));
#11320=CARTESIAN_POINT('Ctrl Pts',(0.521238702715143,-1.17924592340069,
0.7));
#11321=CARTESIAN_POINT('Ctrl Pts',(0.331856371369203,-1.17491202960101,
0.7));
#11322=CARTESIAN_POINT('Origin',(6.87409734069396,-2.22251806091942E-16,
0.7));
#11323=CARTESIAN_POINT('',(0.331856371879032,1.17491202961268,0.7));
#11324=CARTESIAN_POINT('',(0.331856371369201,-0.75,0.7));
#11325=CARTESIAN_POINT('Ctrl Pts',(0.331856371879031,1.17491202961268,0.7));
#11326=CARTESIAN_POINT('Ctrl Pts',(0.521238703055026,1.1792459234085,0.7));
#11327=CARTESIAN_POINT('Ctrl Pts',(0.710620070823648,1.18359647108907,0.7));
#11328=CARTESIAN_POINT('Ctrl Pts',(0.900000000000325,1.18799600975363,0.7));
#11329=CARTESIAN_POINT('Ctrl Pts',(0.297857073289265,1.30643674434242,-1.84041299971672E-5));
#11330=CARTESIAN_POINT('Ctrl Pts',(0.30797052782623,1.29586163793935,0.201769818898405));
#11331=CARTESIAN_POINT('Ctrl Pts',(0.318084017341667,1.28528653282265,0.403558040242397));
#11332=CARTESIAN_POINT('Ctrl Pts',(0.328197542344371,1.27471142901691,0.605346259877786));
#11333=CARTESIAN_POINT('Ctrl Pts',(0.49855879921793,1.31100715551957,-1.17746012218085E-5));
#11334=CARTESIAN_POINT('Ctrl Pts',(0.50835067796626,1.30043204942878,0.201776459067662));
#11335=CARTESIAN_POINT('Ctrl Pts',(0.518142591787414,1.28985694462549,0.403564691103219));
#11336=CARTESIAN_POINT('Ctrl Pts',(0.527934541191015,1.27928184113928,0.60535292148228));
#11337=CARTESIAN_POINT('Ctrl Pts',(0.699273108318888,1.31559634352235,-5.70013621459206E-6));
#11338=CARTESIAN_POINT('Ctrl Pts',(0.708743431409089,1.3050212387088,0.201782543309265));
#11339=CARTESIAN_POINT('Ctrl Pts',(0.718213789762737,1.29444613519316,0.403570785168614));
#11340=CARTESIAN_POINT('Ctrl Pts',(0.727684183892215,1.28387103300524,0.605359025419352));
#11341=CARTESIAN_POINT('Ctrl Pts',(0.9,1.32024227787037,-6.93889390390723E-18));
#11342=CARTESIAN_POINT('Ctrl Pts',(0.909148787559144,1.30966717532775,0.201788252648578));
#11343=CARTESIAN_POINT('Ctrl Pts',(0.918297610668582,1.29909207410301,0.403576503755731));
#11344=CARTESIAN_POINT('Ctrl Pts',(0.927446469845411,1.28851697422136,0.605364753299355));
#11345=CARTESIAN_POINT('',(0.329571806169048,1.2747428754212,0.605346305703265));
#11346=CARTESIAN_POINT('Ctrl Pts',(0.900000001879216,1.28788040990034,0.605337476551906));
#11347=CARTESIAN_POINT('Ctrl Pts',(0.709864288600119,1.28346276435313,0.605340219076093));
#11348=CARTESIAN_POINT('Ctrl Pts',(0.519721397561593,1.27909449722757,0.60534313598158));
#11349=CARTESIAN_POINT('Ctrl Pts',(0.329571806169048,1.2747428754212,0.605346305703265));
#11350=CARTESIAN_POINT('Ctrl Pts',(0.329571806169048,1.2747428754212,0.605346305703265));
#11351=CARTESIAN_POINT('Ctrl Pts',(0.319000553694994,1.28530712634462,0.403564200350134));
#11352=CARTESIAN_POINT('Ctrl Pts',(0.308429283449307,1.29587142805659,0.201782098465301));
#11353=CARTESIAN_POINT('Ctrl Pts',(0.297857995688647,1.306435779838,6.03900610074426E-17));
#11354=CARTESIAN_POINT('Ctrl Pts',(0.331856371369201,1.17491202960101,0.7));
#11355=CARTESIAN_POINT('Ctrl Pts',(0.522011847238246,1.17926361631973,0.7));
#11356=CARTESIAN_POINT('Ctrl Pts',(0.712166351817729,1.18363199317816,0.7));
#11357=CARTESIAN_POINT('Ctrl Pts',(0.902319404079528,1.18804989493878,0.7));
#11358=CARTESIAN_POINT('Ctrl Pts',(0.331195161244124,1.20380556524924,0.7));
#11359=CARTESIAN_POINT('Ctrl Pts',(0.521348914609443,1.20815772874132,0.700000022626678));
#11360=CARTESIAN_POINT('Ctrl Pts',(0.711500071980329,1.21252656425213,0.69999998041973));
#11361=CARTESIAN_POINT('Ctrl Pts',(0.901648075315331,1.21694488185794,0.7));
#11362=CARTESIAN_POINT('Ctrl Pts',(0.330048718948197,1.25390275839508,0.676667306001616));
#11363=CARTESIAN_POINT('Ctrl Pts',(0.52019950796711,1.25825584722226,0.676666267597973));
#11364=CARTESIAN_POINT('Ctrl Pts',(0.710344780071469,1.26262550764723,0.676665329845182));
#11365=CARTESIAN_POINT('Ctrl Pts',(0.900484091294292,1.26704448261357,0.676664431332698));
#11366=CARTESIAN_POINT('Ctrl Pts',(0.329598318905018,1.27358432286302,0.626991130804315));
#11367=CARTESIAN_POINT('Ctrl Pts',(0.519747959090446,1.27793661492756,0.62698844527393));
#11368=CARTESIAN_POINT('Ctrl Pts',(0.709890987426057,1.28230548388611,0.626985988983916));
#11369=CARTESIAN_POINT('Ctrl Pts',(0.900026875890748,1.28672371253673,0.626983665342106));
#11370=CARTESIAN_POINT('Ctrl Pts',(0.329571806169048,1.2747428754212,0.605346305703265));
#11371=CARTESIAN_POINT('Ctrl Pts',(0.519721397561593,1.27909449722757,0.60534313598158));
#11372=CARTESIAN_POINT('Ctrl Pts',(0.709864288600119,1.28346276435313,0.605340219076093));
#11373=CARTESIAN_POINT('Ctrl Pts',(0.900000001879216,1.28788040990034,0.605337476551906));
#11374=CARTESIAN_POINT('Origin',(0.331856371369202,1.17491202960101,0.6));
#11375=CARTESIAN_POINT('Origin',(0.331856371369202,1.17491202960101,0.6));
#11376=CARTESIAN_POINT('Origin',(0.331856371369201,1.17491202960879,0.6));
#11377=CARTESIAN_POINT('Origin',(0.331856371369202,1.17491202960101,0.6));
#11378=CARTESIAN_POINT('Origin',(12.8681436286308,1.83274446434879,0.6));
#11379=CARTESIAN_POINT('Origin',(12.8681436286308,1.83274446434879,0.6));
#11380=CARTESIAN_POINT('',(12.9680065821063,1.83274446434879,0.605233595624294));
#11381=CARTESIAN_POINT('Origin',(12.8681436286308,1.83274446434879,0.6));
#11382=CARTESIAN_POINT('Origin',(12.8681436286308,1.83274446434879,0.6));
#11383=CARTESIAN_POINT('Origin',(0.331856371369201,-1.17491202960101,0.6));
#11384=CARTESIAN_POINT('Origin',(0.331856371369201,-1.17491202960101,0.6));
#11385=CARTESIAN_POINT('Origin',(0.331856371369201,-1.17491202960101,0.6));
#11386=CARTESIAN_POINT('Origin',(0.331856371369201,-0.75,0.6));
#11387=CARTESIAN_POINT('Ctrl Pts',(0.297750759617602,-1.30654294555098,
-0.00204689530870639));
#11388=CARTESIAN_POINT('Ctrl Pts',(0.308357792853923,-1.29594287152607,
0.200417501569666));
#11389=CARTESIAN_POINT('Ctrl Pts',(0.318964808457496,-1.28534284790734,
0.40288190189057));
#11390=CARTESIAN_POINT('Ctrl Pts',(0.329571806169048,-1.2747428754212,0.605346305703266));
#11391=CARTESIAN_POINT('Ctrl Pts',(0.268364475985512,-1.30579334864515,
-0.000546070465277405));
#11392=CARTESIAN_POINT('Ctrl Pts',(0.278972236061358,-1.29519218153762,
0.201918231169276));
#11393=CARTESIAN_POINT('Ctrl Pts',(0.289579970322816,-1.28459115545203,
0.404382541571378));
#11394=CARTESIAN_POINT('Ctrl Pts',(0.300187702091134,-1.27399007937578,
0.606846849214128));
#11395=CARTESIAN_POINT('Ctrl Pts',(0.217994620733579,-1.28028753054242,
0.000758348866131992));
#11396=CARTESIAN_POINT('Ctrl Pts',(0.228604439653725,-1.26968580576698,
0.203222517770204));
#11397=CARTESIAN_POINT('Ctrl Pts',(0.239214264875756,-1.259084092946,0.405686686833815));
#11398=CARTESIAN_POINT('Ctrl Pts',(0.24982407554016,-1.24848245399652,0.608150860486448));
#11399=CARTESIAN_POINT('Ctrl Pts',(0.200221638751335,-1.22875730734246,
-0.00100806500432267));
#11400=CARTESIAN_POINT('Ctrl Pts',(0.210832346469089,-1.21815680658782,
0.201456130081263));
#11401=CARTESIAN_POINT('Ctrl Pts',(0.221443027663539,-1.20755634130466,
0.403920328365886));
#11402=CARTESIAN_POINT('Ctrl Pts',(0.232053735729819,-1.1969559383274,0.606384528499152));
#11403=CARTESIAN_POINT('Ctrl Pts',(0.200161316008396,-1.20671181983024,
-0.00215909150772397));
#11404=CARTESIAN_POINT('Ctrl Pts',(0.21077201649647,-1.19611183845239,0.200305134857769));
#11405=CARTESIAN_POINT('Ctrl Pts',(0.221382717124246,-1.18551190812967,
0.402769363888924));
#11406=CARTESIAN_POINT('Ctrl Pts',(0.231993417893744,-1.17491202960101,
0.605233595624295));
#11407=CARTESIAN_POINT('Origin',(12.8681436286308,-1.83274446434879,0.6));
#11408=CARTESIAN_POINT('',(12.9680065821063,-1.83274446434879,0.605233595624295));
#11409=CARTESIAN_POINT('Origin',(12.8681436286308,-1.83274446434879,0.6));
#11410=CARTESIAN_POINT('Origin',(12.8681436286308,-1.83274446434879,0.6));
#11411=CARTESIAN_POINT('Origin',(12.8681436286308,1.1,0.6));
#11412=CARTESIAN_POINT('',(12.9680065821063,1.1,0.605233595624295));
#11413=CARTESIAN_POINT('Ctrl Pts',(12.9998428721614,-1.86475648739599,-0.00223900654757928));
#11414=CARTESIAN_POINT('Ctrl Pts',(12.9892307746816,-1.85408610159386,0.200251876006837));
#11415=CARTESIAN_POINT('Ctrl Pts',(12.9786186779927,-1.84341542867022,0.402742743472647));
#11416=CARTESIAN_POINT('Ctrl Pts',(12.9680065821063,-1.83274446434879,0.605233595624296));
#11417=CARTESIAN_POINT('Ctrl Pts',(12.9997989521977,-1.88070362541494,-0.00140096371806573));
#11418=CARTESIAN_POINT('Ctrl Pts',(12.9891868560404,-1.87003481788623,0.2010900171988));
#11419=CARTESIAN_POINT('Ctrl Pts',(12.9785747412344,-1.85936572080465,0.403580981971657));
#11420=CARTESIAN_POINT('Ctrl Pts',(12.967962646681,-1.84869634914788,0.606071933479074));
#11421=CARTESIAN_POINT('Ctrl Pts',(12.9919061104719,-1.91252097257855,-0.00013797468654593));
#11422=CARTESIAN_POINT('Ctrl Pts',(12.9812924311808,-1.9018552985481,0.202353118580234));
#11423=CARTESIAN_POINT('Ctrl Pts',(12.970678744243,-1.89118929884075,0.404844194499128));
#11424=CARTESIAN_POINT('Ctrl Pts',(12.9600650516023,-1.88052308923615,0.607335259545336));
#11425=CARTESIAN_POINT('Ctrl Pts',(12.9539932318948,-1.95585643963679,0.000158685530800887));
#11426=CARTESIAN_POINT('Ctrl Pts',(12.9433725220626,-1.94519261899951,0.202649549046396));
#11427=CARTESIAN_POINT('Ctrl Pts',(12.9327517623504,-1.93452853669393,0.40514039680648));
#11428=CARTESIAN_POINT('Ctrl Pts',(12.9221309734579,-1.92386419524738,0.607631230057729));
#11429=CARTESIAN_POINT('Ctrl Pts',(12.9129235702791,-1.96658826742031,-0.00142816374191492));
#11430=CARTESIAN_POINT('Ctrl Pts',(12.9022969271978,-1.95592037993921,0.201062184830579));
#11431=CARTESIAN_POINT('Ctrl Pts',(12.891670251582,-1.94525202616943,0.403552507423554));
#11432=CARTESIAN_POINT('Ctrl Pts',(12.8810434760214,-1.93458357684419,0.60604282089977));
#11433=CARTESIAN_POINT('Ctrl Pts',(12.8891437477602,-1.96405813112492,-0.00280773857265357));
#11434=CARTESIAN_POINT('Ctrl Pts',(12.8785151960038,-1.95338599020215,0.199682283294402));
#11435=CARTESIAN_POINT('Ctrl Pts',(12.8678865709412,-1.94271355010484,0.402172286243574));
#11436=CARTESIAN_POINT('Ctrl Pts',(12.8572578715866,-1.93204080633595,0.604662269998931));
#11437=CARTESIAN_POINT('Ctrl Pts',(12.9997255308004,-1.86463850151065,-4.9439619065339E-17));
#11438=CARTESIAN_POINT('Ctrl Pts',(12.9891525471135,-1.85400744222428,0.201744546927532));
#11439=CARTESIAN_POINT('Ctrl Pts',(12.9785795642115,-1.84337609791338,0.403489078876654));
#11440=CARTESIAN_POINT('Ctrl Pts',(12.9680065821063,-1.83274446434879,0.605233595624296));
#11441=CARTESIAN_POINT('Ctrl Pts',(12.8891409639924,1.96405533594058,-0.00275470357795049));
#11442=CARTESIAN_POINT('Ctrl Pts',(12.8785133401458,1.95338412669368,0.199717639954231));
#11443=CARTESIAN_POINT('Ctrl Pts',(12.8678856430057,1.9427126183241,0.402189964571813));
#11444=CARTESIAN_POINT('Ctrl Pts',(12.8572578715866,1.93204080633595,0.604662269998929));
#11445=CARTESIAN_POINT('Ctrl Pts',(12.9049941793403,1.96574209420267,-0.00183498696757459));
#11446=CARTESIAN_POINT('Ctrl Pts',(12.8943678341644,1.95507368670196,0.20063757283533));
#11447=CARTESIAN_POINT('Ctrl Pts',(12.8837414238008,1.94440496992476,0.403110113573296));
#11448=CARTESIAN_POINT('Ctrl Pts',(12.8731149412098,1.93373598667478,0.605582637266155));
#11449=CARTESIAN_POINT('Ctrl Pts',(12.9374710816243,1.9613461313261,-0.000364592700753267));
#11450=CARTESIAN_POINT('Ctrl Pts',(12.9268487371951,1.95068187676899,0.202108391447626));
#11451=CARTESIAN_POINT('Ctrl Pts',(12.9162262930262,1.94001732715406,0.404581355450702));
#11452=CARTESIAN_POINT('Ctrl Pts',(12.9056038462248,1.92935253789361,0.607054307450502));
#11453=CARTESIAN_POINT('Ctrl Pts',(12.9846523118271,1.92834870343354,0.000369250346899581));
#11454=CARTESIAN_POINT('Ctrl Pts',(12.974038022963,1.91768545846127,0.202842678583437));
#11455=CARTESIAN_POINT('Ctrl Pts',(12.9634237233674,1.90702194269714,0.405316092420461));
#11456=CARTESIAN_POINT('Ctrl Pts',(12.9528094065597,1.89635817580376,0.607789492622546));
#11457=CARTESIAN_POINT('Ctrl Pts',(12.9997742127558,1.88867440031858,-0.000928907044737527));
#11458=CARTESIAN_POINT('Ctrl Pts',(12.9891630904765,1.8780073281596,0.201544447891303));
#11459=CARTESIAN_POINT('Ctrl Pts',(12.9785517991681,1.86733992038445,0.404017776344753));
#11460=CARTESIAN_POINT('Ctrl Pts',(12.9679406789684,1.85667229154743,0.606491102406462));
#11461=CARTESIAN_POINT('Ctrl Pts',(12.9998400927033,1.86475369267134,-0.00218597132744988));
#11462=CARTESIAN_POINT('Ctrl Pts',(12.9892289217097,1.85408423839396,0.200287232817622));
#11463=CARTESIAN_POINT('Ctrl Pts',(12.9786177515068,1.84341449704483,0.402760421876702));
#11464=CARTESIAN_POINT('Ctrl Pts',(12.9680065821063,1.83274446434879,0.605233595624294));
#11465=CARTESIAN_POINT('Ctrl Pts',(12.9680065821063,1.83274446434879,0.605233595624294));
#11466=CARTESIAN_POINT('Ctrl Pts',(12.9785795642115,1.84337609791338,0.403489078876654));
#11467=CARTESIAN_POINT('Ctrl Pts',(12.9891525471135,1.85400744222428,0.201744546927532));
#11468=CARTESIAN_POINT('Ctrl Pts',(12.9997255308004,1.86463850151065,1.86916454536501E-16));
#11469=CARTESIAN_POINT('Ctrl Pts',(12.6,1.80383022254432,0.7));
#11470=CARTESIAN_POINT('Ctrl Pts',(12.6893984576578,1.8133105623702,0.7));
#11471=CARTESIAN_POINT('Ctrl Pts',(12.7787800350189,1.82294762441299,0.7));
#11472=CARTESIAN_POINT('Ctrl Pts',(12.8681436286308,1.83274446434879,0.7));
#11473=CARTESIAN_POINT('Ctrl Pts',(12.5969393303222,1.83269196733649,0.7));
#11474=CARTESIAN_POINT('Ctrl Pts',(12.686303642571,1.84217134991284,0.700000098415946));
#11475=CARTESIAN_POINT('Ctrl Pts',(12.7756511334299,1.85180730951691,0.699999896874207));
#11476=CARTESIAN_POINT('Ctrl Pts',(12.8649798835675,1.86160311979107,0.7));
#11477=CARTESIAN_POINT('Ctrl Pts',(12.5916356538948,1.88270499442536,0.67643906321291));
#11478=CARTESIAN_POINT('Ctrl Pts',(12.6809412203008,1.89218243450198,0.676434576658958));
#11479=CARTESIAN_POINT('Ctrl Pts',(12.7702288461642,1.90181652272411,0.676430055978541));
#11480=CARTESIAN_POINT('Ctrl Pts',(12.8594976525144,1.91161025179704,0.676425356750174));
#11481=CARTESIAN_POINT('Ctrl Pts',(12.58957419749,1.90214427893475,0.626447702441804));
#11482=CARTESIAN_POINT('Ctrl Pts',(12.6788572782758,1.91161594713488,0.626436135819418));
#11483=CARTESIAN_POINT('Ctrl Pts',(12.7681225846323,1.92124403769089,0.626424372515079));
#11484=CARTESIAN_POINT('Ctrl Pts',(12.8573684983393,1.93103170500986,0.626412260100396));
#11485=CARTESIAN_POINT('Ctrl Pts',(12.5894662143615,1.90316254677271,0.604704117718382));
#11486=CARTESIAN_POINT('Ctrl Pts',(12.6787484942245,1.91263121188366,0.60469048808123));
#11487=CARTESIAN_POINT('Ctrl Pts',(12.7680127446979,1.92225628370762,0.604676541242762));
#11488=CARTESIAN_POINT('Ctrl Pts',(12.8572578715866,1.93204080633595,0.60466226999893));
#11489=CARTESIAN_POINT('Ctrl Pts',(0.200160815981423,1.20671231935208,-0.00216863259073552));
#11490=CARTESIAN_POINT('Ctrl Pts',(0.21077168314515,1.19611217146534,0.200298774135678));
#11491=CARTESIAN_POINT('Ctrl Pts',(0.221382550448584,1.18551207463533,0.402766183527835));
#11492=CARTESIAN_POINT('Ctrl Pts',(0.231993417893744,1.17491202960101,0.605233595624295));
#11493=CARTESIAN_POINT('Ctrl Pts',(0.200241246305444,1.23610630273461,-0.000633930584249493));
#11494=CARTESIAN_POINT('Ctrl Pts',(0.210852138766318,1.22550544237485,0.201833432539687));
#11495=CARTESIAN_POINT('Ctrl Pts',(0.221462948692539,1.21490467236247,0.404300804744641));
#11496=CARTESIAN_POINT('Ctrl Pts',(0.232073841675177,1.20430390790287,0.60676817279077));
#11497=CARTESIAN_POINT('Ctrl Pts',(0.224595236946023,1.28704077752974,0.000756396927320467));
#11498=CARTESIAN_POINT('Ctrl Pts',(0.235204871724134,1.27643877611169,0.203223757667495));
#11499=CARTESIAN_POINT('Ctrl Pts',(0.245814524913363,1.26583679641595,0.405691118453359));
#11500=CARTESIAN_POINT('Ctrl Pts',(0.256424148042823,1.25523487973404,0.608158484046399));
#11501=CARTESIAN_POINT('Ctrl Pts',(0.275710547013829,1.30598124743532,-0.000930817763883136));
#11502=CARTESIAN_POINT('Ctrl Pts',(0.286318282165364,1.29538020346814,0.201536689442792));
#11503=CARTESIAN_POINT('Ctrl Pts',(0.296926023167072,1.2847792285374,0.404004199876323));
#11504=CARTESIAN_POINT('Ctrl Pts',(0.307533728110612,1.27417827838713,0.606471713336412));
#11505=CARTESIAN_POINT('Ctrl Pts',(0.297750259763447,1.30654344507719,-0.0020564363997533));
#11506=CARTESIAN_POINT('Ctrl Pts',(0.308357459618374,1.29594320454196,0.200411140842193));
#11507=CARTESIAN_POINT('Ctrl Pts',(0.318964641840002,1.28534301441448,0.402878721526778));
#11508=CARTESIAN_POINT('Ctrl Pts',(0.329571806169048,1.2747428754212,0.605346305703265));
#11509=CARTESIAN_POINT('Origin',(13.0002740930491,2.2,-0.0104671912485888));
#11510=CARTESIAN_POINT('Origin',(0.331856371369202,1.17491202960101,0.6));
#11511=CARTESIAN_POINT('',(0.331856371879032,1.17491202961268,0.9));
#11512=CARTESIAN_POINT('',(0.0322675109428289,1.17491202960101,0.615700786872883));
#11513=CARTESIAN_POINT('Origin',(0.331856371369201,1.17491202962433,0.6));
#11514=CARTESIAN_POINT('',(0.325002675768741,1.47440456706157,0.616038917109795));
#11515=CARTESIAN_POINT('Origin',(0.331856371369202,1.17491202960101,0.6));
#11516=CARTESIAN_POINT('Origin',(0.331856371369201,1.17491202960101,0.6));
#11517=CARTESIAN_POINT('Origin',(12.8681436286308,1.83274446434879,0.6));
#11518=CARTESIAN_POINT('',(12.8681436286308,1.83274446434879,0.9));
#11519=CARTESIAN_POINT('',(12.8354863574981,2.13063349031027,0.613986809996789));
#11520=CARTESIAN_POINT('Origin',(12.8681436286308,1.83274446434879,0.6));
#11521=CARTESIAN_POINT('',(13.1677324890572,1.83274446434879,0.615700786872883));
#11522=CARTESIAN_POINT('Origin',(12.8681436286308,1.83274446434879,0.6));
#11523=CARTESIAN_POINT('Origin',(12.8681436286308,1.83274446434879,0.6));
#11524=CARTESIAN_POINT('Origin',(0.331856371369201,-1.17491202960101,0.6));
#11525=CARTESIAN_POINT('',(0.331856371369201,-1.17491202962433,0.9));
#11526=CARTESIAN_POINT('',(0.325002675768743,-1.47440456706157,0.616038917109795));
#11527=CARTESIAN_POINT('Origin',(0.331856371879032,-1.17491202961268,0.6));
#11528=CARTESIAN_POINT('',(0.0322675109428289,-1.17491202960101,0.615700786872884));
#11529=CARTESIAN_POINT('Origin',(0.331856371369201,-1.17491202960101,0.6));
#11530=CARTESIAN_POINT('Origin',(0.331856371369201,-1.17491202960101,0.6));
#11531=CARTESIAN_POINT('Origin',(0.331856371369201,-0.75,0.6));
#11532=CARTESIAN_POINT('',(0.0322675109428289,-0.75,0.615700786872883));
#11533=CARTESIAN_POINT('',(0.331856371369201,-0.75,0.9));
#11534=CARTESIAN_POINT('Ctrl Pts',(0.292429673212981,-1.5069793045954,-0.00614074949474724));
#11535=CARTESIAN_POINT('Ctrl Pts',(0.303287396789886,-1.49612100698918,
0.201252467440773));
#11536=CARTESIAN_POINT('Ctrl Pts',(0.314145064588525,-1.48526276089333,
0.408645689616972));
#11537=CARTESIAN_POINT('Ctrl Pts',(0.325002675768741,-1.47440456706157,
0.616038917109795));
#11538=CARTESIAN_POINT('Ctrl Pts',(0.204270663953122,-1.50473074636003,
-0.00163825452108868));
#11539=CARTESIAN_POINT('Ctrl Pts',(0.215130619942527,-1.49386909866124,
0.205754670272474));
#11540=CARTESIAN_POINT('Ctrl Pts',(0.225990497234893,-1.48300775583971,
0.413147615201549));
#11541=CARTESIAN_POINT('Ctrl Pts',(0.236850363534999,-1.47214617892531,
0.620540547642382));
#11542=CARTESIAN_POINT('Ctrl Pts',(0.0531014592841718,-1.42831231122466,
0.00228331220810075));
#11543=CARTESIAN_POINT('Ctrl Pts',(0.0639677431943945,-1.41744892560022,
0.209675827753147));
#11544=CARTESIAN_POINT('Ctrl Pts',(0.0748340498672138,-1.40658548887187,
0.417068339030394));
#11545=CARTESIAN_POINT('Ctrl Pts',(0.0857003072238147,-1.3957221574093,
0.624460858243749));
#11546=CARTESIAN_POINT('Ctrl Pts',(-0.000158492362241063,-1.27362248439808,
-0.0030242144278773));
#11547=CARTESIAN_POINT('Ctrl Pts',(0.0107105192099893,-1.2627628846508,
0.204368383073371));
#11548=CARTESIAN_POINT('Ctrl Pts',(0.0215794523842628,-1.25190326350425,
0.411760983371354));
#11549=CARTESIAN_POINT('Ctrl Pts',(0.0324484644510542,-1.24104375578019,
0.619153585497454));
#11550=CARTESIAN_POINT('Ctrl Pts',(-0.000339460947516079,-1.20748590713937,
-0.00647730073969574));
#11551=CARTESIAN_POINT('Ctrl Pts',(0.0105295295353408,-1.19662789414299,
0.200915392321314));
#11552=CARTESIAN_POINT('Ctrl Pts',(0.0213985201647323,-1.18576993469886,
0.408308088178364));
#11553=CARTESIAN_POINT('Ctrl Pts',(0.032267510942829,-1.17491202960101,
0.615700786872884));
#11554=CARTESIAN_POINT('Ctrl Pts',(0.292751161823634,-1.50665779898694,
4.33680868994202E-17));
#11555=CARTESIAN_POINT('Ctrl Pts',(0.30350172143464,-1.49590667092872,0.205346300540216));
#11556=CARTESIAN_POINT('Ctrl Pts',(0.314252226354851,-1.48515559337638,
0.410692606218909));
#11557=CARTESIAN_POINT('Ctrl Pts',(0.325002675768741,-1.47440456706157,
0.616038917109795));
#11558=CARTESIAN_POINT('Ctrl Pts',(0.032267510942829,-1.17491202960101,
0.615700786872884));
#11559=CARTESIAN_POINT('Ctrl Pts',(0.021511673816962,-1.18565689645617,
0.410467188483275));
#11560=CARTESIAN_POINT('Ctrl Pts',(0.0107558368367201,-1.19640181653194,
0.205233592872363));
#11561=CARTESIAN_POINT('Ctrl Pts',(-2.19605150036939E-16,-1.20714678905882,
1.11889664200504E-16));
#11562=CARTESIAN_POINT('Origin',(12.8681436286308,-1.83274446434879,0.6));
#11563=CARTESIAN_POINT('',(13.1677324890572,-1.83274446434879,0.615700786872883));
#11564=CARTESIAN_POINT('',(12.8354863574981,-2.13063349031027,0.613986809996789));
#11565=CARTESIAN_POINT('Origin',(12.8681436286308,-1.83274446434879,0.6));
#11566=CARTESIAN_POINT('',(12.8681436286308,-1.83274446434879,0.9));
#11567=CARTESIAN_POINT('Origin',(12.8681436286308,-1.83274446434879,0.6));
#11568=CARTESIAN_POINT('Origin',(12.8681436286308,-1.83274446434879,0.6));
#11569=CARTESIAN_POINT('Origin',(12.8681436286308,1.1,0.6));
#11570=CARTESIAN_POINT('',(13.1677324890572,1.1,0.615700786872883));
#11571=CARTESIAN_POINT('',(12.8681436286308,1.1,0.9));
#11572=CARTESIAN_POINT('Ctrl Pts',(12.8681436286308,-1.83274446434879,0.9));
#11573=CARTESIAN_POINT('Ctrl Pts',(11.0848390724976,-1.63724259846481,0.9));
#11574=CARTESIAN_POINT('Ctrl Pts',(6.90843812479705,-1.33014681916253,0.9));
#11575=CARTESIAN_POINT('Ctrl Pts',(2.72316671642812,-1.22963564084767,0.9));
#11576=CARTESIAN_POINT('Ctrl Pts',(0.331856371369203,-1.17491202960101,
0.9));
#11577=CARTESIAN_POINT('Ctrl Pts',(12.8586523934408,-1.91932043067563,0.9));
#11578=CARTESIAN_POINT('Ctrl Pts',(11.0774332085042,-1.7238803779394,0.89999435405169));
#11579=CARTESIAN_POINT('Ctrl Pts',(6.90489492800773,-1.41683381760594,0.900002805573959));
#11580=CARTESIAN_POINT('Ctrl Pts',(2.72111811994416,-1.31633797570969,0.90000078069347));
#11581=CARTESIAN_POINT('Ctrl Pts',(0.329872740993971,-1.26159263654569,
0.9));
#11582=CARTESIAN_POINT('Ctrl Pts',(12.8422006781022,-2.06938763738452,0.829321796184829));
#11583=CARTESIAN_POINT('Ctrl Pts',(11.0645720435655,-1.87407163985848,0.829602081442736));
#11584=CARTESIAN_POINT('Ctrl Pts',(6.89876476423634,-1.56711486110062,0.829953500700133));
#11585=CARTESIAN_POINT('Ctrl Pts',(2.71756729604702,-1.46664725828863,0.829952661937692));
#11586=CARTESIAN_POINT('Ctrl Pts',(0.326433810179884,-1.41186690836963,
0.829991693349937));
#11587=CARTESIAN_POINT('Ctrl Pts',(12.8358182377562,-2.12760618633201,0.679236780301187));
#11588=CARTESIAN_POINT('Ctrl Pts',(11.0595580661442,-1.93265366192027,0.679962478070753));
#11589=CARTESIAN_POINT('Ctrl Pts',(6.89634818471837,-1.62613750062048,0.680874066334139));
#11590=CARTESIAN_POINT('Ctrl Pts',(2.71617242066404,-1.52567909229178,0.680871998075852));
#11591=CARTESIAN_POINT('Ctrl Pts',(0.325082213976654,-1.47092890938704,
0.680973392412944));
#11592=CARTESIAN_POINT('Ctrl Pts',(12.8354863574981,-2.13063349031027,0.613986809996789));
#11593=CARTESIAN_POINT('Ctrl Pts',(11.0592740266891,-1.93586902238569,0.614841183901826));
#11594=CARTESIAN_POINT('Ctrl Pts',(6.89620783868867,-1.62958780289117,0.615922665333222));
#11595=CARTESIAN_POINT('Ctrl Pts',(2.71609101918193,-1.52912950204849,0.615919334096661));
#11596=CARTESIAN_POINT('Ctrl Pts',(0.325002675768742,-1.47440456706157,
0.616038917109795));
#11597=CARTESIAN_POINT('Ctrl Pts',(0.325002675768742,-1.47440456706157,
0.616038917109795));
#11598=CARTESIAN_POINT('Ctrl Pts',(2.71609101918193,-1.52912950204849,0.615919334096661));
#11599=CARTESIAN_POINT('Ctrl Pts',(6.89620783868867,-1.62958780289117,0.615922665333222));
#11600=CARTESIAN_POINT('Ctrl Pts',(11.0592740266891,-1.93586902238569,0.614841183901826));
#11601=CARTESIAN_POINT('Ctrl Pts',(12.8354863574981,-2.13063349031027,0.613986809996789));
#11602=CARTESIAN_POINT('Ctrl Pts',(12.8681436286308,-1.83274446434879,0.9));
#11603=CARTESIAN_POINT('Ctrl Pts',(11.0848390724976,-1.63724259846481,0.9));
#11604=CARTESIAN_POINT('Ctrl Pts',(6.90843812479705,-1.33014681916253,0.9));
#11605=CARTESIAN_POINT('Ctrl Pts',(2.72316671642812,-1.22963564084767,0.9));
#11606=CARTESIAN_POINT('Ctrl Pts',(0.331856371369203,-1.17491202960101,
0.9));
#11607=CARTESIAN_POINT('Ctrl Pts',(13.2003520234216,-1.86554403325358,-0.00671700702553119));
#11608=CARTESIAN_POINT('Ctrl Pts',(13.1894788444661,-1.85461114646479,0.200755606855839));
#11609=CARTESIAN_POINT('Ctrl Pts',(13.1786056663403,-1.84367795836273,0.40822820490283));
#11610=CARTESIAN_POINT('Ctrl Pts',(13.1677324890572,-1.83274446434879,0.615700786872884));
#11611=CARTESIAN_POINT('Ctrl Pts',(13.200220264666,-1.91338509859121,-0.00420290020003313));
#11612=CARTESIAN_POINT('Ctrl Pts',(13.1893470894366,-1.90245705934317,0.203270015787334));
#11613=CARTESIAN_POINT('Ctrl Pts',(13.1784738563058,-1.89152871992859,0.410742913234898));
#11614=CARTESIAN_POINT('Ctrl Pts',(13.1676006827814,-1.88060011874606,0.61821580043722));
#11615=CARTESIAN_POINT('Ctrl Pts',(13.1765676699515,-2.00888806967359,-0.000409897060868941));
#11616=CARTESIAN_POINT('Ctrl Pts',(13.1656896254949,-1.99796966505382,0.207063364242462));
#11617=CARTESIAN_POINT('Ctrl Pts',(13.1548115799789,-1.98705090404177,0.414536607525659));
#11618=CARTESIAN_POINT('Ctrl Pts',(13.1439334900924,-1.97613202744891,0.622009843787749));
#11619=CARTESIAN_POINT('Ctrl Pts',(13.0627995670833,-2.13884429305335,0.000475886042502645));
#11620=CARTESIAN_POINT('Ctrl Pts',(13.0518999280859,-2.12793157960824,0.207948441605934));
#11621=CARTESIAN_POINT('Ctrl Pts',(13.041000104914,-2.11701865581933,0.415420978499924));
#11622=CARTESIAN_POINT('Ctrl Pts',(13.0301002136907,-2.10610551685206,0.62289350259018));
#11623=CARTESIAN_POINT('Ctrl Pts',(12.9395973356642,-2.17103883395928,-0.00428435975826336));
#11624=CARTESIAN_POINT('Ctrl Pts',(12.9286794517625,-2.16011362679945,0.203186612960554));
#11625=CARTESIAN_POINT('Ctrl Pts',(12.9177614752639,-2.14918756369419,0.410657536673191));
#11626=CARTESIAN_POINT('Ctrl Pts',(12.9068431708026,-2.13826180183499,0.618128462699307));
#11627=CARTESIAN_POINT('Ctrl Pts',(12.8682582931239,-2.16344935299393,-0.00842301254802964));
#11628=CARTESIAN_POINT('Ctrl Pts',(12.857334548107,-2.15251107312608,0.1990469563258));
#11629=CARTESIAN_POINT('Ctrl Pts',(12.8464105706338,-2.1415724540018,0.406516897309109));
#11630=CARTESIAN_POINT('Ctrl Pts',(12.8354863574981,-2.13063349031027,0.61398680999679));
#11631=CARTESIAN_POINT('Ctrl Pts',(13.2,-1.86519007666192,-2.60208521396521E-17));
#11632=CARTESIAN_POINT('Ctrl Pts',(13.1892441622028,-1.85437516893481,0.20523361119958));
#11633=CARTESIAN_POINT('Ctrl Pts',(13.1784883252177,-1.84355996631422,0.410467206902138));
#11634=CARTESIAN_POINT('Ctrl Pts',(13.1677324890572,-1.83274446434879,0.615700786872884));
#11635=CARTESIAN_POINT('Ctrl Pts',(12.8354863574981,-2.13063349031027,0.61398680999679));
#11636=CARTESIAN_POINT('Ctrl Pts',(12.8462627343229,-2.14142441807303,0.409324567403199));
#11637=CARTESIAN_POINT('Ctrl Pts',(12.8570388818204,-2.15221501053143,0.204662297274642));
#11638=CARTESIAN_POINT('Ctrl Pts',(12.8678148030684,-2.16300527278357,2.15973072759112E-16));
#11639=CARTESIAN_POINT('Ctrl Pts',(12.868249917342,2.16344096606744,-0.0082639349430893));
#11640=CARTESIAN_POINT('Ctrl Pts',(12.8573289641336,2.15250548166836,0.19915300804817));
#11641=CARTESIAN_POINT('Ctrl Pts',(12.8464077785869,2.14156965818488,0.406569923163064));
#11642=CARTESIAN_POINT('Ctrl Pts',(12.8354863574981,2.13063349031027,0.613986809996789));
#11643=CARTESIAN_POINT('Ctrl Pts',(12.9158092820513,2.16850062662823,-0.00550483257449158));
#11644=CARTESIAN_POINT('Ctrl Pts',(12.9048922561706,2.15757374897544,0.201912774743134));
#11645=CARTESIAN_POINT('Ctrl Pts',(12.8939750281693,2.14664650750606,0.409330354360154));
#11646=CARTESIAN_POINT('Ctrl Pts',(12.8830575663678,2.13571903132675,0.616747911798467));
#11647=CARTESIAN_POINT('Ctrl Pts',(13.0132876381743,2.15534286385676,-0.00108956416640176));
#11648=CARTESIAN_POINT('Ctrl Pts',(13.002382910411,2.14442874534411,0.206329347217122));
#11649=CARTESIAN_POINT('Ctrl Pts',(12.9914779109393,2.13351435475356,0.413748232116966));
#11650=CARTESIAN_POINT('Ctrl Pts',(12.9805728576194,2.12259976690609,0.621167106093357));
#11651=CARTESIAN_POINT('Ctrl Pts',(13.1547834649542,2.05631410774027,0.001107541479323));
#11652=CARTESIAN_POINT('Ctrl Pts',(13.1439034803964,2.04540309863889,0.208527817346591));
#11653=CARTESIAN_POINT('Ctrl Pts',(13.1330234810862,2.03449182132921,0.415948079627069));
#11654=CARTESIAN_POINT('Ctrl Pts',(13.1221434051731,2.0235803832085,0.623368331037722));
#11655=CARTESIAN_POINT('Ctrl Pts',(13.2001460482598,1.93729725403583,-0.00278676680844524));
#11656=CARTESIAN_POINT('Ctrl Pts',(13.1892758011844,1.92637447722781,0.204633283810596));
#11657=CARTESIAN_POINT('Ctrl Pts',(13.1784050234814,1.91545126126866,0.412053283701094));
#11658=CARTESIAN_POINT('Ctrl Pts',(13.1675347796435,1.9045279459447,0.619473307219386));
#11659=CARTESIAN_POINT('Ctrl Pts',(13.2003436864113,1.86553565046225,-0.00655792739252892));
#11660=CARTESIAN_POINT('Ctrl Pts',(13.1894732864596,1.85460555778322,0.200861659936414));
#11661=CARTESIAN_POINT('Ctrl Pts',(13.1786028873373,1.84367516394377,0.408281231439009));
#11662=CARTESIAN_POINT('Ctrl Pts',(13.1677324890572,1.83274446434879,0.615700786872883));
#11663=CARTESIAN_POINT('Ctrl Pts',(12.8678148030684,2.16300527278357,-3.77302356024956E-17));
#11664=CARTESIAN_POINT('Ctrl Pts',(12.8570388818204,2.15221501053142,0.204662297274639));
#11665=CARTESIAN_POINT('Ctrl Pts',(12.8462627343229,2.14142441807303,0.409324567403198));
#11666=CARTESIAN_POINT('Ctrl Pts',(12.8354863574981,2.13063349031027,0.613986809996789));
#11667=CARTESIAN_POINT('Ctrl Pts',(13.1677324890572,1.83274446434879,0.615700786872883));
#11668=CARTESIAN_POINT('Ctrl Pts',(13.1784883252177,1.84355996631422,0.410467206902138));
#11669=CARTESIAN_POINT('Ctrl Pts',(13.1892441622028,1.85437516893481,0.20523361119958));
#11670=CARTESIAN_POINT('Ctrl Pts',(13.2,1.86519007666192,9.4542429440736E-17));
#11671=CARTESIAN_POINT('Ctrl Pts',(0.3318563713692,1.17491202960101,0.9));
#11672=CARTESIAN_POINT('Ctrl Pts',(2.72316671642811,1.22963564084767,0.9));
#11673=CARTESIAN_POINT('Ctrl Pts',(6.90843812479704,1.33014681916253,0.9));
#11674=CARTESIAN_POINT('Ctrl Pts',(11.0848390724976,1.63724259846481,0.9));
#11675=CARTESIAN_POINT('Ctrl Pts',(12.8681436286308,1.83274446434879,0.9));
#11676=CARTESIAN_POINT('Ctrl Pts',(0.329872740993969,1.26159263654569,0.9));
#11677=CARTESIAN_POINT('Ctrl Pts',(2.72111811994415,1.31633797570969,0.90000078069347));
#11678=CARTESIAN_POINT('Ctrl Pts',(6.90489492800774,1.41683381760594,0.90000280557396));
#11679=CARTESIAN_POINT('Ctrl Pts',(11.0774332085042,1.7238803779394,0.89999435405169));
#11680=CARTESIAN_POINT('Ctrl Pts',(12.8586523934408,1.91932043067563,0.9));
#11681=CARTESIAN_POINT('Ctrl Pts',(0.326433810179882,1.41186690836963,0.829991693349937));
#11682=CARTESIAN_POINT('Ctrl Pts',(2.71756729604703,1.46664725828863,0.829952661937692));
#11683=CARTESIAN_POINT('Ctrl Pts',(6.89876476423633,1.56711486110062,0.829953500700133));
#11684=CARTESIAN_POINT('Ctrl Pts',(11.0645720435655,1.87407163985848,0.829602081442736));
#11685=CARTESIAN_POINT('Ctrl Pts',(12.8422006781022,2.06938763738452,0.829321796184828));
#11686=CARTESIAN_POINT('Ctrl Pts',(0.325082213976652,1.47092890938703,0.680973392412944));
#11687=CARTESIAN_POINT('Ctrl Pts',(2.71617242066403,1.52567909229178,0.680871998075852));
#11688=CARTESIAN_POINT('Ctrl Pts',(6.89634818471838,1.62613750062048,0.680874066334139));
#11689=CARTESIAN_POINT('Ctrl Pts',(11.0595580661442,1.93265366192027,0.679962478070753));
#11690=CARTESIAN_POINT('Ctrl Pts',(12.8358182377562,2.12760618633201,0.679236780301187));
#11691=CARTESIAN_POINT('Ctrl Pts',(0.32500267576874,1.47440456706157,0.616038917109795));
#11692=CARTESIAN_POINT('Ctrl Pts',(2.71609101918192,1.52912950204849,0.615919334096661));
#11693=CARTESIAN_POINT('Ctrl Pts',(6.89620783868868,1.62958780289117,0.615922665333222));
#11694=CARTESIAN_POINT('Ctrl Pts',(11.0592740266891,1.93586902238569,0.614841183901826));
#11695=CARTESIAN_POINT('Ctrl Pts',(12.8354863574981,2.13063349031027,0.613986809996789));
#11696=CARTESIAN_POINT('Ctrl Pts',(12.8354863574981,2.13063349031027,0.613986809996789));
#11697=CARTESIAN_POINT('Ctrl Pts',(11.0592740266891,1.93586902238569,0.614841183901826));
#11698=CARTESIAN_POINT('Ctrl Pts',(6.89620783868868,1.62958780289117,0.615922665333222));
#11699=CARTESIAN_POINT('Ctrl Pts',(2.71609101918192,1.52912950204849,0.615919334096661));
#11700=CARTESIAN_POINT('Ctrl Pts',(0.32500267576874,1.47440456706157,0.616038917109795));
#11701=CARTESIAN_POINT('Ctrl Pts',(0.331856371879031,1.17491202961268,0.900000000000001));
#11702=CARTESIAN_POINT('Ctrl Pts',(2.72316671676804,1.22963564085583,0.9));
#11703=CARTESIAN_POINT('Ctrl Pts',(6.90843812496665,1.330146819175,0.9));
#11704=CARTESIAN_POINT('Ctrl Pts',(11.0848390724976,1.63724259846481,0.9));
#11705=CARTESIAN_POINT('Ctrl Pts',(12.8681436286308,1.83274446434879,0.9));
#11706=CARTESIAN_POINT('Ctrl Pts',(-0.00034095850043725,1.20748740317979,
-0.0065058757516861));
#11707=CARTESIAN_POINT('Ctrl Pts',(0.0105285311667133,1.19662889149835,
0.200896342313063));
#11708=CARTESIAN_POINT('Ctrl Pts',(0.0213980209804115,1.18577043337405,
0.408298563174108));
#11709=CARTESIAN_POINT('Ctrl Pts',(0.0322675109428289,1.17491202960101,
0.615700786872884));
#11710=CARTESIAN_POINT('Ctrl Pts',(-9.96670524854573E-5,1.295669506487,
-0.00190176065173685));
#11711=CARTESIAN_POINT('Ctrl Pts',(0.0107698931059531,1.28480880908357,
0.205500324005663));
#11712=CARTESIAN_POINT('Ctrl Pts',(0.0216392211477595,1.27394827585187,
0.412902429485043));
#11713=CARTESIAN_POINT('Ctrl Pts',(0.0325087822871292,1.26308766450658,
0.62030451837231));
#11714=CARTESIAN_POINT('Ctrl Pts',(0.0728623575603101,1.44853010213391,
0.00227745497540766));
#11715=CARTESIAN_POINT('Ctrl Pts',(0.0837280751164453,1.43766588856392,
0.209679530627308));
#11716=CARTESIAN_POINT('Ctrl Pts',(0.0945938325013454,1.42680163888532,
0.41708160190494));
#11717=CARTESIAN_POINT('Ctrl Pts',(0.105459512942901,1.41593747613444,0.624483681552028));
#11718=CARTESIAN_POINT('Ctrl Pts',(0.226308920038025,1.50529438233544,-0.00279245331904538));
#11719=CARTESIAN_POINT('Ctrl Pts',(0.237168779176494,1.4944331215396,0.204610074087555));
#11720=CARTESIAN_POINT('Ctrl Pts',(0.248028678199983,1.48357195724705,0.412012604182119));
#11721=CARTESIAN_POINT('Ctrl Pts',(0.258888441593434,1.47271077595937,0.619415140009235));
#11722=CARTESIAN_POINT('Ctrl Pts',(0.292428177212438,1.50698080067503,-0.00616932457891824));
#11723=CARTESIAN_POINT('Ctrl Pts',(0.303286399461314,1.49612200437087,0.201233417384176));
#11724=CARTESIAN_POINT('Ctrl Pts',(0.314144565926839,1.48526325958177,0.408636164588429));
#11725=CARTESIAN_POINT('Ctrl Pts',(0.325002675768741,1.47440456706157,0.616038917109795));
#11726=CARTESIAN_POINT('Ctrl Pts',(1.62630325872826E-19,1.20714678905882,
-9.93129189996722E-17));
#11727=CARTESIAN_POINT('Ctrl Pts',(0.0107558368367203,1.19640181653194,
0.205233592872363));
#11728=CARTESIAN_POINT('Ctrl Pts',(0.0215116738169619,1.18565689645617,
0.410467188483274));
#11729=CARTESIAN_POINT('Ctrl Pts',(0.0322675109428289,1.17491202960101,
0.615700786872884));
#11730=CARTESIAN_POINT('Ctrl Pts',(0.325002675768741,1.47440456706157,0.616038917109795));
#11731=CARTESIAN_POINT('Ctrl Pts',(0.314252226354851,1.48515559337638,0.410692606218907));
#11732=CARTESIAN_POINT('Ctrl Pts',(0.30350172143464,1.49590667092872,0.205346300540215));
#11733=CARTESIAN_POINT('Ctrl Pts',(0.292751161823635,1.50665779898694,-1.27502175484295E-16));
#11734=CARTESIAN_POINT('Ctrl Pts',(12.8678148030684,-2.16300527278356,0.));
#11735=CARTESIAN_POINT('Ctrl Pts',(12.8575947095063,-2.15224352891768,0.205346305703265));
#11736=CARTESIAN_POINT('Ctrl Pts',(12.8473746159443,-2.14148178505179,0.41069261140653));
#11737=CARTESIAN_POINT('Ctrl Pts',(12.8371545223823,-2.13072004118591,0.616038917109795));
#11738=CARTESIAN_POINT('Ctrl Pts',(8.67612692265345,-1.70561506876628,0.));
#11739=CARTESIAN_POINT('Ctrl Pts',(8.67274165808153,-1.69485332490039,0.205346305703265));
#11740=CARTESIAN_POINT('Ctrl Pts',(8.66935639350961,-1.68409158103451,0.41069261140653));
#11741=CARTESIAN_POINT('Ctrl Pts',(8.6659711289377,-1.67332983716862,0.616038917109795));
#11742=CARTESIAN_POINT('Ctrl Pts',(4.48443904223854,-1.60211086545473,0.));
#11743=CARTESIAN_POINT('Ctrl Pts',(4.48788860665674,-1.59134912158884,0.205346305703265));
#11744=CARTESIAN_POINT('Ctrl Pts',(4.49133817107494,-1.58058737772296,0.41069261140653));
#11745=CARTESIAN_POINT('Ctrl Pts',(4.49478773549313,-1.56982563385707,0.616038917109795));
#11746=CARTESIAN_POINT('Ctrl Pts',(0.292751161823634,-1.50665779898694,
0.));
#11747=CARTESIAN_POINT('Ctrl Pts',(0.303035555231945,-1.49589605512106,
0.205346305703265));
#11748=CARTESIAN_POINT('Ctrl Pts',(0.313319948640256,-1.48513431125517,
0.41069261140653));
#11749=CARTESIAN_POINT('Ctrl Pts',(0.323604342048567,-1.47437256738929,
0.616038917109795));
#11750=CARTESIAN_POINT('Origin',(0.,-1.5,0.));
#11751=CARTESIAN_POINT('Origin',(6.87409734069396,-2.22044604925031E-16,
0.9));
#11752=CARTESIAN_POINT('Ctrl Pts',(0.292751161823634,1.50665779898694,0.));
#11753=CARTESIAN_POINT('Ctrl Pts',(0.303035555231945,1.49589605512106,0.205346305703265));
#11754=CARTESIAN_POINT('Ctrl Pts',(0.313319948640256,1.48513431125517,0.41069261140653));
#11755=CARTESIAN_POINT('Ctrl Pts',(0.323604342048567,1.47437256738929,0.616038917109795));
#11756=CARTESIAN_POINT('Ctrl Pts',(4.48443904223854,1.60211086545473,0.));
#11757=CARTESIAN_POINT('Ctrl Pts',(4.48788860665674,1.59134912158884,0.205346305703265));
#11758=CARTESIAN_POINT('Ctrl Pts',(4.49133817107493,1.58058737772296,0.41069261140653));
#11759=CARTESIAN_POINT('Ctrl Pts',(4.49478773549313,1.56982563385707,0.616038917109795));
#11760=CARTESIAN_POINT('Ctrl Pts',(8.67612692265345,1.70561506876628,0.));
#11761=CARTESIAN_POINT('Ctrl Pts',(8.67274165808153,1.69485332490039,0.205346305703265));
#11762=CARTESIAN_POINT('Ctrl Pts',(8.66935639350961,1.68409158103451,0.41069261140653));
#11763=CARTESIAN_POINT('Ctrl Pts',(8.66597112893769,1.67332983716862,0.616038917109795));
#11764=CARTESIAN_POINT('Ctrl Pts',(12.8678148030684,2.16300527278356,0.));
#11765=CARTESIAN_POINT('Ctrl Pts',(12.8575947095063,2.15224352891768,0.205346305703265));
#11766=CARTESIAN_POINT('Ctrl Pts',(12.8473746159443,2.14148178505179,0.41069261140653));
#11767=CARTESIAN_POINT('Ctrl Pts',(12.8371545223823,2.13072004118591,0.616038917109795));
#11768=CARTESIAN_POINT('Origin',(13.2,2.2,0.));
#19599=UNCERTAINTY_MEASURE_WITH_UNIT(LENGTH_MEASURE(0.001),#19619,
'DISTANCE_ACCURACY_VALUE',
'Maximum model space distance between geometric entities at asserted c
onnectivities');
#19605=UNCERTAINTY_MEASURE_WITH_UNIT(LENGTH_MEASURE(0.001),#19619,
'DISTANCE_ACCURACY_VALUE',
'Maximum model space distance between geometric entities at asserted c
onnectivities');
#19612=(
GEOMETRIC_REPRESENTATION_CONTEXT(3)
GLOBAL_UNCERTAINTY_ASSIGNED_CONTEXT((#19599))
GLOBAL_UNIT_ASSIGNED_CONTEXT((#19619,#19621,#19622))
REPRESENTATION_CONTEXT('','3D')
);
#19618=(
GEOMETRIC_REPRESENTATION_CONTEXT(3)
GLOBAL_UNCERTAINTY_ASSIGNED_CONTEXT((#19605))
GLOBAL_UNIT_ASSIGNED_CONTEXT((#19619,#19621,#19622))
REPRESENTATION_CONTEXT('','3D')
);
#19619=(
LENGTH_UNIT()
NAMED_UNIT(*)
SI_UNIT(.CENTI.,.METRE.)
);
#19621=(
NAMED_UNIT(*)
PLANE_ANGLE_UNIT()
SI_UNIT($,.RADIAN.)
);
#19622=(
NAMED_UNIT(*)
SI_UNIT($,.STERADIAN.)
SOLID_ANGLE_UNIT()
);
#19629=SHAPE_DEFINITION_REPRESENTATION(#19641,#19669);
#19641=PRODUCT_DEFINITION_SHAPE('',$,#19682);
#19669=SHAPE_REPRESENTATION('',(#7373),#19612);
#19675=PRODUCT_DEFINITION_CONTEXT('part definition',#19713,'design');
#19682=PRODUCT_DEFINITION('2026-11-10-01-34-59-955',
'Upper structural shell',#19694,#19675);
#19694=PRODUCT_DEFINITION_FORMATION('',$,#19721);
#19713=APPLICATION_CONTEXT(
'Core Data for Automotive Mechanical Design Process');
#19714=PRODUCT_CONTEXT('part definition',#19713,'mechanical');
#19721=PRODUCT('2026-11-10-01-34-59-955','Upper structural shell',$,(#19714));
#19731=PRESENTATION_STYLE_ASSIGNMENT((#19739));
#19739=SURFACE_STYLE_USAGE(.BOTH.,#19747);
#19747=SURFACE_SIDE_STYLE('',(#19755));
#19755=SURFACE_STYLE_FILL_AREA(#19763);
#19763=FILL_AREA_STYLE('Structural dark blue',(#19771));
#19771=FILL_AREA_STYLE_COLOUR('Structural dark blue',#19779);
#19779=COLOUR_RGB('Structural dark blue',0.0901960784313725,0.270588235294118,
0.513725490196078);
ENDSEC;
END-ISO-10303-21;
